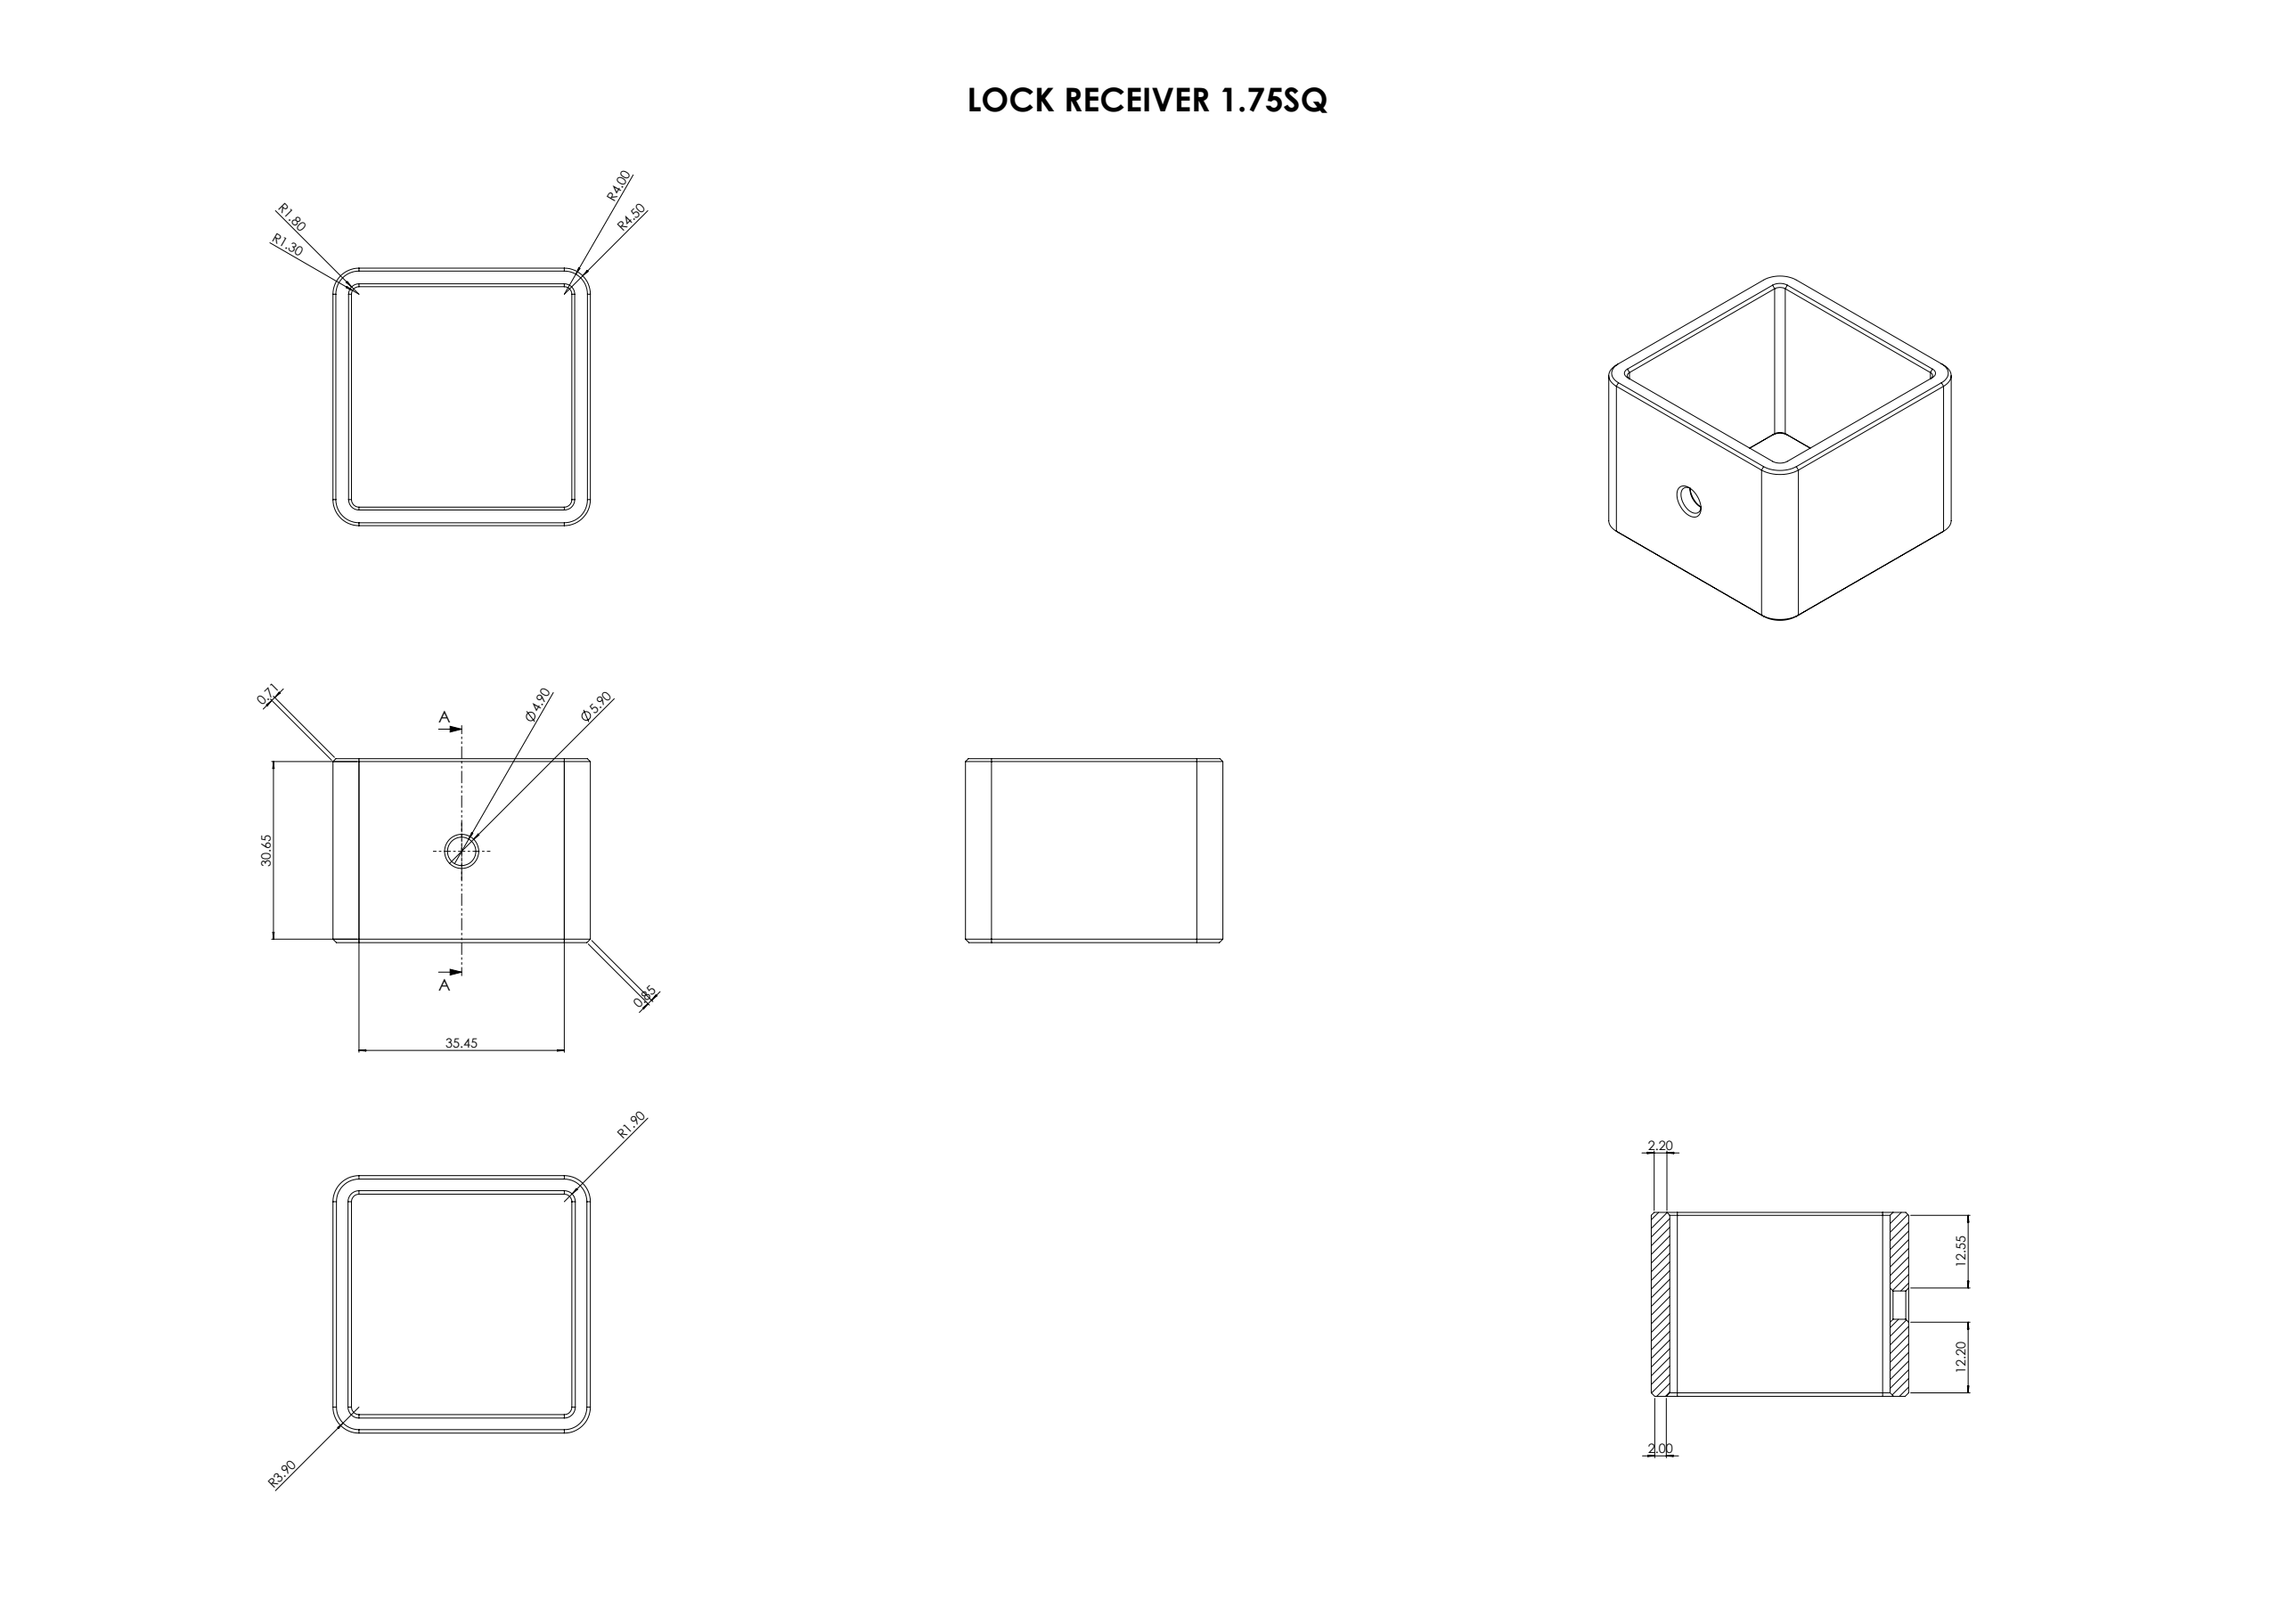
ISO-10303-21;
HEADER;
/* Generated by software containing ST-Developer
 * from STEP Tools, Inc. (www.steptools.com) 
 */

FILE_DESCRIPTION(
/* description */ (''),
/* implementation_level */ '2;1');

FILE_NAME(
/* name */ '04_Lock_Receiver_1.75sq.step',
/* time_stamp */ '2026-10-25T01:30:15-07:00',
/* author */ (''),
/* organization */ (''),
/* preprocessor_version */ 'ST-DEVELOPER v20.2',
/* originating_system */ 'Autodesk Translation Framework v15.15.0.0',
/* authorisation */ '');

FILE_SCHEMA (('AUTOMOTIVE_DESIGN { 1 0 10303 214 3 1 1 }'));
ENDSEC;

DATA;
#10=MECHANICAL_DESIGN_GEOMETRIC_PRESENTATION_REPRESENTATION('',(#566),#32309);
#538=SHAPE_REPRESENTATION_RELATIONSHIP('SRR','None',#32365,#552);
#552=ADVANCED_BREP_SHAPE_REPRESENTATION('',(#580),#32298);
#566=STYLED_ITEM('',(#32516),#580);
#580=MANIFOLD_SOLID_BREP('Body1',#13807);
#595=FACE_BOUND('',#2179,.T.);
#596=FACE_BOUND('',#2182,.T.);
#597=FACE_BOUND('',#2196,.T.);
#598=FACE_BOUND('',#2218,.T.);
#676=CYLINDRICAL_SURFACE('',#14118,2.45);
#677=CYLINDRICAL_SURFACE('',#14140,1.30000000000001);
#678=CYLINDRICAL_SURFACE('',#14143,1.30000000000001);
#679=CYLINDRICAL_SURFACE('',#14164,4.50000000000001);
#680=CYLINDRICAL_SURFACE('',#14167,4.50000000000001);
#681=CYLINDRICAL_SURFACE('',#14198,1.3);
#682=CYLINDRICAL_SURFACE('',#14199,1.3);
#683=CYLINDRICAL_SURFACE('',#14201,4.5);
#684=CYLINDRICAL_SURFACE('',#14203,4.5);
#819=CIRCLE('',#14116,2.95);
#820=CIRCLE('',#14117,2.45);
#821=CIRCLE('',#14119,2.45);
#822=CIRCLE('',#14122,2.95);
#823=CIRCLE('',#14126,1.80000000000001);
#824=CIRCLE('',#14127,1.30000000000001);
#825=CIRCLE('',#14130,1.80000000000001);
#826=CIRCLE('',#14131,1.30000000000001);
#827=CIRCLE('',#14134,1.8);
#828=CIRCLE('',#14135,1.3);
#829=CIRCLE('',#14138,1.8);
#830=CIRCLE('',#14139,1.3);
#831=CIRCLE('',#14141,1.30000000000001);
#832=CIRCLE('',#14144,1.30000000000001);
#833=CIRCLE('',#14147,4.00000000000001);
#834=CIRCLE('',#14148,4.00000000000001);
#835=CIRCLE('',#14149,4.);
#836=CIRCLE('',#14150,4.);
#837=CIRCLE('',#14152,4.50000000000001);
#838=CIRCLE('',#14155,4.50000000000001);
#839=CIRCLE('',#14158,4.5);
#840=CIRCLE('',#14161,4.5);
#841=CIRCLE('',#14165,4.50000000000001);
#842=CIRCLE('',#14168,4.50000000000001);
#843=CIRCLE('',#14171,3.90000000000001);
#844=CIRCLE('',#14174,3.90000000000001);
#845=CIRCLE('',#14177,3.9);
#846=CIRCLE('',#14178,4.5);
#847=CIRCLE('',#14181,3.9);
#848=CIRCLE('',#14182,4.5);
#849=CIRCLE('',#14184,1.90000000000001);
#850=CIRCLE('',#14185,1.9);
#851=CIRCLE('',#14186,1.9);
#852=CIRCLE('',#14187,1.90000000000001);
#853=CIRCLE('',#14192,1.3);
#854=CIRCLE('',#14195,1.3);
#1117=CONICAL_SURFACE('',#14115,2.7,0.785398163397451);
#1118=CONICAL_SURFACE('',#14121,2.7,0.785398163397448);
#1119=CONICAL_SURFACE('',#14125,1.55000000000001,0.785398163397447);
#1120=CONICAL_SURFACE('',#14129,1.55000000000001,0.785398163397447);
#1121=CONICAL_SURFACE('',#14133,1.55,0.785398163397449);
#1122=CONICAL_SURFACE('',#14137,1.55,0.785398163397448);
#1123=CONICAL_SURFACE('',#14151,4.25000000000001,0.785398163397448);
#1124=CONICAL_SURFACE('',#14154,4.25000000000001,0.785398163397448);
#1125=CONICAL_SURFACE('',#14157,4.25,0.785398163397448);
#1126=CONICAL_SURFACE('',#14160,4.25,0.785398163397448);
#1127=CONICAL_SURFACE('',#14170,4.20000000000001,0.78539816339745);
#1128=CONICAL_SURFACE('',#14173,4.20000000000001,0.78539816339745);
#1129=CONICAL_SURFACE('',#14176,4.2,0.785398163397449);
#1130=CONICAL_SURFACE('',#14180,4.2,0.785398163397449);
#1131=CONICAL_SURFACE('',#14189,1.60000000000001,0.785398163397449);
#1132=CONICAL_SURFACE('',#14191,1.6,0.785398163397447);
#1133=CONICAL_SURFACE('',#14194,1.6,0.785398163397448);
#1134=CONICAL_SURFACE('',#14197,1.60000000000001,0.78539816339745);
#1373=FACE_OUTER_BOUND('',#2176,.T.);
#1374=FACE_OUTER_BOUND('',#2177,.T.);
#1375=FACE_OUTER_BOUND('',#2178,.T.);
#1376=FACE_OUTER_BOUND('',#2180,.T.);
#1377=FACE_OUTER_BOUND('',#2181,.T.);
#1378=FACE_OUTER_BOUND('',#2183,.T.);
#1379=FACE_OUTER_BOUND('',#2184,.T.);
#1380=FACE_OUTER_BOUND('',#2185,.T.);
#1381=FACE_OUTER_BOUND('',#2186,.T.);
#1382=FACE_OUTER_BOUND('',#2187,.T.);
#1383=FACE_OUTER_BOUND('',#2188,.T.);
#1384=FACE_OUTER_BOUND('',#2189,.T.);
#1385=FACE_OUTER_BOUND('',#2190,.T.);
#1386=FACE_OUTER_BOUND('',#2191,.T.);
#1387=FACE_OUTER_BOUND('',#2192,.T.);
#1388=FACE_OUTER_BOUND('',#2193,.T.);
#1389=FACE_OUTER_BOUND('',#2194,.T.);
#1390=FACE_OUTER_BOUND('',#2195,.T.);
#1391=FACE_OUTER_BOUND('',#2197,.T.);
#1392=FACE_OUTER_BOUND('',#2198,.T.);
#1393=FACE_OUTER_BOUND('',#2199,.T.);
#1394=FACE_OUTER_BOUND('',#2200,.T.);
#1395=FACE_OUTER_BOUND('',#2201,.T.);
#1396=FACE_OUTER_BOUND('',#2202,.T.);
#1397=FACE_OUTER_BOUND('',#2203,.T.);
#1398=FACE_OUTER_BOUND('',#2204,.T.);
#1399=FACE_OUTER_BOUND('',#2205,.T.);
#1400=FACE_OUTER_BOUND('',#2206,.T.);
#1401=FACE_OUTER_BOUND('',#2207,.T.);
#1402=FACE_OUTER_BOUND('',#2208,.T.);
#1403=FACE_OUTER_BOUND('',#2209,.T.);
#1404=FACE_OUTER_BOUND('',#2210,.T.);
#1405=FACE_OUTER_BOUND('',#2211,.T.);
#1406=FACE_OUTER_BOUND('',#2212,.T.);
#1407=FACE_OUTER_BOUND('',#2213,.T.);
#1408=FACE_OUTER_BOUND('',#2214,.T.);
#1409=FACE_OUTER_BOUND('',#2215,.T.);
#1410=FACE_OUTER_BOUND('',#2216,.T.);
#1411=FACE_OUTER_BOUND('',#2217,.T.);
#1412=FACE_OUTER_BOUND('',#2219,.T.);
#1413=FACE_OUTER_BOUND('',#2220,.T.);
#1414=FACE_OUTER_BOUND('',#2221,.T.);
#1415=FACE_OUTER_BOUND('',#2222,.T.);
#1416=FACE_OUTER_BOUND('',#2223,.T.);
#1417=FACE_OUTER_BOUND('',#2224,.T.);
#1418=FACE_OUTER_BOUND('',#2225,.T.);
#1419=FACE_OUTER_BOUND('',#2226,.T.);
#1420=FACE_OUTER_BOUND('',#2227,.T.);
#1421=FACE_OUTER_BOUND('',#2228,.T.);
#1422=FACE_OUTER_BOUND('',#2229,.T.);
#1423=FACE_OUTER_BOUND('',#2230,.T.);
#1424=FACE_OUTER_BOUND('',#2231,.T.);
#1425=FACE_OUTER_BOUND('',#2232,.T.);
#2176=EDGE_LOOP('',(#9317,#9318,#9319,#9320));
#2177=EDGE_LOOP('',(#9321,#9322,#9323,#9324));
#2178=EDGE_LOOP('',(#9325,#9326,#9327,#9328));
#2179=EDGE_LOOP('',(#9329));
#2180=EDGE_LOOP('',(#9330,#9331,#9332,#9333));
#2181=EDGE_LOOP('',(#9334,#9335,#9336,#9337));
#2182=EDGE_LOOP('',(#9338));
#2183=EDGE_LOOP('',(#9339,#9340,#9341,#9342));
#2184=EDGE_LOOP('',(#9343,#9344,#9345,#9346));
#2185=EDGE_LOOP('',(#9347,#9348,#9349,#9350));
#2186=EDGE_LOOP('',(#9351,#9352,#9353,#9354));
#2187=EDGE_LOOP('',(#9355,#9356,#9357,#9358));
#2188=EDGE_LOOP('',(#9359,#9360,#9361,#9362));
#2189=EDGE_LOOP('',(#9363,#9364,#9365,#9366));
#2190=EDGE_LOOP('',(#9367,#9368,#9369,#9370));
#2191=EDGE_LOOP('',(#9371,#9372,#9373,#9374));
#2192=EDGE_LOOP('',(#9375,#9376,#9377,#9378));
#2193=EDGE_LOOP('',(#9379,#9380,#9381,#9382));
#2194=EDGE_LOOP('',(#9383,#9384,#9385,#9386));
#2195=EDGE_LOOP('',(#9387,#9388,#9389,#9390,#9391,#9392,#9393,#9394));
#2196=EDGE_LOOP('',(#9395,#9396,#9397,#9398,#9399,#9400,#9401,#9402));
#2197=EDGE_LOOP('',(#9403,#9404,#9405,#9406));
#2198=EDGE_LOOP('',(#9407,#9408,#9409,#9410));
#2199=EDGE_LOOP('',(#9411,#9412,#9413,#9414));
#2200=EDGE_LOOP('',(#9415,#9416,#9417,#9418));
#2201=EDGE_LOOP('',(#9419,#9420,#9421,#9422));
#2202=EDGE_LOOP('',(#9423,#9424,#9425,#9426));
#2203=EDGE_LOOP('',(#9427,#9428,#9429,#9430));
#2204=EDGE_LOOP('',(#9431,#9432,#9433,#9434));
#2205=EDGE_LOOP('',(#9435,#9436,#9437,#9438));
#2206=EDGE_LOOP('',(#9439,#9440,#9441,#9442));
#2207=EDGE_LOOP('',(#9443,#9444,#9445,#9446));
#2208=EDGE_LOOP('',(#9447,#9448,#9449,#9450));
#2209=EDGE_LOOP('',(#9451,#9452,#9453,#9454));
#2210=EDGE_LOOP('',(#9455,#9456,#9457,#9458));
#2211=EDGE_LOOP('',(#9459,#9460,#9461,#9462));
#2212=EDGE_LOOP('',(#9463,#9464,#9465,#9466));
#2213=EDGE_LOOP('',(#9467,#9468,#9469,#9470));
#2214=EDGE_LOOP('',(#9471,#9472,#9473,#9474));
#2215=EDGE_LOOP('',(#9475,#9476,#9477,#9478));
#2216=EDGE_LOOP('',(#9479,#9480,#9481,#9482));
#2217=EDGE_LOOP('',(#9483,#9484,#9485,#9486,#9487,#9488,#9489,#9490));
#2218=EDGE_LOOP('',(#9491,#9492,#9493,#9494,#9495,#9496,#9497,#9498));
#2219=EDGE_LOOP('',(#9499,#9500,#9501,#9502));
#2220=EDGE_LOOP('',(#9503,#9504,#9505,#9506));
#2221=EDGE_LOOP('',(#9507,#9508,#9509,#9510));
#2222=EDGE_LOOP('',(#9511,#9512,#9513,#9514));
#2223=EDGE_LOOP('',(#9515,#9516,#9517,#9518));
#2224=EDGE_LOOP('',(#9519,#9520,#9521,#9522));
#2225=EDGE_LOOP('',(#9523,#9524,#9525,#9526));
#2226=EDGE_LOOP('',(#9527,#9528,#9529,#9530));
#2227=EDGE_LOOP('',(#9531,#9532,#9533,#9534));
#2228=EDGE_LOOP('',(#9535,#9536,#9537,#9538));
#2229=EDGE_LOOP('',(#9539,#9540,#9541,#9542));
#2230=EDGE_LOOP('',(#9543,#9544,#9545,#9546));
#2231=EDGE_LOOP('',(#9547,#9548,#9549,#9550));
#2232=EDGE_LOOP('',(#9551,#9552,#9553,#9554));
#3065=LINE('',#21996,#4376);
#3066=LINE('',#22000,#4377);
#3067=LINE('',#22005,#4378);
#3068=LINE('',#22007,#4379);
#3069=LINE('',#22009,#4380);
#3070=LINE('',#22010,#4381);
#3071=LINE('',#22014,#4382);
#3072=LINE('',#22018,#4383);
#3073=LINE('',#22020,#4384);
#3074=LINE('',#22022,#4385);
#3075=LINE('',#22023,#4386);
#3076=LINE('',#22027,#4387);
#3077=LINE('',#22029,#4388);
#3078=LINE('',#22031,#4389);
#3079=LINE('',#22032,#4390);
#3080=LINE('',#22036,#4391);
#3081=LINE('',#22042,#4392);
#3082=LINE('',#22043,#4393);
#3083=LINE('',#22044,#4394);
#3084=LINE('',#22047,#4395);
#3085=LINE('',#22052,#4396);
#3086=LINE('',#22053,#4397);
#3087=LINE('',#22057,#4398);
#3088=LINE('',#22063,#4399);
#3089=LINE('',#22064,#4400);
#3090=LINE('',#22065,#4401);
#3091=LINE('',#22071,#4402);
#3092=LINE('',#22075,#4403);
#3093=LINE('',#22076,#4404);
#3094=LINE('',#22079,#4405);
#3095=LINE('',#22083,#4406);
#3096=LINE('',#22084,#4407);
#3097=LINE('',#22090,#4408);
#3098=LINE('',#22094,#4409);
#3099=LINE('',#22098,#4410);
#3100=LINE('',#22101,#4411);
#3101=LINE('',#22104,#4412);
#3102=LINE('',#22105,#4413);
#3103=LINE('',#22109,#4414);
#3104=LINE('',#22110,#4415);
#3105=LINE('',#22113,#4416);
#3106=LINE('',#22117,#4417);
#3107=LINE('',#22118,#4418);
#3108=LINE('',#22121,#4419);
#3109=LINE('',#22125,#4420);
#3110=LINE('',#22126,#4421);
#3111=LINE('',#22128,#4422);
#3112=LINE('',#22133,#4423);
#3113=LINE('',#22135,#4424);
#3114=LINE('',#22136,#4425);
#3115=LINE('',#22139,#4426);
#3116=LINE('',#22143,#4427);
#3117=LINE('',#22144,#4428);
#3118=LINE('',#22149,#4429);
#3119=LINE('',#22151,#4430);
#3120=LINE('',#22152,#4431);
#3121=LINE('',#22155,#4432);
#3122=LINE('',#22159,#4433);
#3123=LINE('',#22160,#4434);
#3124=LINE('',#22163,#4435);
#3125=LINE('',#22167,#4436);
#3126=LINE('',#22168,#4437);
#3127=LINE('',#22172,#4438);
#3128=LINE('',#22178,#4439);
#3129=LINE('',#22179,#4440);
#3130=LINE('',#22180,#4441);
#3131=LINE('',#22187,#4442);
#3132=LINE('',#22191,#4443);
#3133=LINE('',#22195,#4444);
#3134=LINE('',#22199,#4445);
#3135=LINE('',#22202,#4446);
#3136=LINE('',#22203,#4447);
#3137=LINE('',#22205,#4448);
#3138=LINE('',#22207,#4449);
#3139=LINE('',#22210,#4450);
#3140=LINE('',#22214,#4451);
#3141=LINE('',#22215,#4452);
#3142=LINE('',#22217,#4453);
#3143=LINE('',#22220,#4454);
#3144=LINE('',#22223,#4455);
#3145=LINE('',#22225,#4456);
#3146=LINE('',#22228,#4457);
#3147=LINE('',#22230,#4458);
#4376=VECTOR('',#15461,2.7);
#4377=VECTOR('',#15466,2.45);
#4378=VECTOR('',#15471,10.);
#4379=VECTOR('',#15472,10.);
#4380=VECTOR('',#15473,10.);
#4381=VECTOR('',#15474,10.);
#4382=VECTOR('',#15479,2.7);
#4383=VECTOR('',#15482,10.);
#4384=VECTOR('',#15483,10.);
#4385=VECTOR('',#15484,10.);
#4386=VECTOR('',#15485,10.);
#4387=VECTOR('',#15488,10.);
#4388=VECTOR('',#15489,10.);
#4389=VECTOR('',#15490,10.);
#4390=VECTOR('',#15491,10.);
#4391=VECTOR('',#15494,10.);
#4392=VECTOR('',#15501,10.);
#4393=VECTOR('',#15502,10.);
#4394=VECTOR('',#15503,10.);
#4395=VECTOR('',#15506,10.);
#4396=VECTOR('',#15513,10.);
#4397=VECTOR('',#15514,10.);
#4398=VECTOR('',#15517,10.);
#4399=VECTOR('',#15524,10.);
#4400=VECTOR('',#15525,10.);
#4401=VECTOR('',#15526,10.);
#4402=VECTOR('',#15535,10.);
#4403=VECTOR('',#15540,10.);
#4404=VECTOR('',#15541,10.);
#4405=VECTOR('',#15544,10.);
#4406=VECTOR('',#15549,10.);
#4407=VECTOR('',#15550,10.);
#4408=VECTOR('',#15555,10.);
#4409=VECTOR('',#15558,10.);
#4410=VECTOR('',#15561,10.);
#4411=VECTOR('',#15564,10.);
#4412=VECTOR('',#15567,10.);
#4413=VECTOR('',#15568,10.);
#4414=VECTOR('',#15573,10.);
#4415=VECTOR('',#15574,10.);
#4416=VECTOR('',#15577,10.);
#4417=VECTOR('',#15582,10.);
#4418=VECTOR('',#15583,10.);
#4419=VECTOR('',#15586,10.);
#4420=VECTOR('',#15591,10.);
#4421=VECTOR('',#15592,10.);
#4422=VECTOR('',#15595,10.);
#4423=VECTOR('',#15602,10.);
#4424=VECTOR('',#15603,10.);
#4425=VECTOR('',#15604,10.);
#4426=VECTOR('',#15607,10.);
#4427=VECTOR('',#15612,10.);
#4428=VECTOR('',#15613,10.);
#4429=VECTOR('',#15620,10.);
#4430=VECTOR('',#15621,10.);
#4431=VECTOR('',#15622,10.);
#4432=VECTOR('',#15625,10.);
#4433=VECTOR('',#15630,10.);
#4434=VECTOR('',#15631,10.);
#4435=VECTOR('',#15634,10.);
#4436=VECTOR('',#15639,10.);
#4437=VECTOR('',#15640,10.);
#4438=VECTOR('',#15643,10.);
#4439=VECTOR('',#15650,10.);
#4440=VECTOR('',#15651,10.);
#4441=VECTOR('',#15652,10.);
#4442=VECTOR('',#15661,10.);
#4443=VECTOR('',#15664,10.);
#4444=VECTOR('',#15667,10.);
#4445=VECTOR('',#15670,10.);
#4446=VECTOR('',#15675,10.);
#4447=VECTOR('',#15676,10.);
#4448=VECTOR('',#15679,10.);
#4449=VECTOR('',#15682,10.);
#4450=VECTOR('',#15685,10.);
#4451=VECTOR('',#15690,10.);
#4452=VECTOR('',#15691,10.);
#4453=VECTOR('',#15694,10.);
#4454=VECTOR('',#15699,10.);
#4455=VECTOR('',#15704,10.);
#4456=VECTOR('',#15707,10.);
#4457=VECTOR('',#15712,10.);
#4458=VECTOR('',#15715,10.);
#5712=VERTEX_POINT('',#21993);
#5713=VERTEX_POINT('',#21995);
#5714=VERTEX_POINT('',#21999);
#5715=VERTEX_POINT('',#22003);
#5716=VERTEX_POINT('',#22004);
#5717=VERTEX_POINT('',#22006);
#5718=VERTEX_POINT('',#22008);
#5719=VERTEX_POINT('',#22012);
#5720=VERTEX_POINT('',#22016);
#5721=VERTEX_POINT('',#22017);
#5722=VERTEX_POINT('',#22019);
#5723=VERTEX_POINT('',#22021);
#5724=VERTEX_POINT('',#22025);
#5725=VERTEX_POINT('',#22026);
#5726=VERTEX_POINT('',#22028);
#5727=VERTEX_POINT('',#22030);
#5728=VERTEX_POINT('',#22034);
#5729=VERTEX_POINT('',#22035);
#5730=VERTEX_POINT('',#22040);
#5731=VERTEX_POINT('',#22041);
#5732=VERTEX_POINT('',#22046);
#5733=VERTEX_POINT('',#22051);
#5734=VERTEX_POINT('',#22055);
#5735=VERTEX_POINT('',#22056);
#5736=VERTEX_POINT('',#22061);
#5737=VERTEX_POINT('',#22062);
#5738=VERTEX_POINT('',#22070);
#5739=VERTEX_POINT('',#22074);
#5740=VERTEX_POINT('',#22078);
#5741=VERTEX_POINT('',#22082);
#5742=VERTEX_POINT('',#22086);
#5743=VERTEX_POINT('',#22087);
#5744=VERTEX_POINT('',#22089);
#5745=VERTEX_POINT('',#22091);
#5746=VERTEX_POINT('',#22093);
#5747=VERTEX_POINT('',#22095);
#5748=VERTEX_POINT('',#22097);
#5749=VERTEX_POINT('',#22099);
#5750=VERTEX_POINT('',#22103);
#5751=VERTEX_POINT('',#22108);
#5752=VERTEX_POINT('',#22112);
#5753=VERTEX_POINT('',#22116);
#5754=VERTEX_POINT('',#22120);
#5755=VERTEX_POINT('',#22124);
#5756=VERTEX_POINT('',#22132);
#5757=VERTEX_POINT('',#22134);
#5758=VERTEX_POINT('',#22138);
#5759=VERTEX_POINT('',#22142);
#5760=VERTEX_POINT('',#22148);
#5761=VERTEX_POINT('',#22150);
#5762=VERTEX_POINT('',#22154);
#5763=VERTEX_POINT('',#22158);
#5764=VERTEX_POINT('',#22162);
#5765=VERTEX_POINT('',#22166);
#5766=VERTEX_POINT('',#22170);
#5767=VERTEX_POINT('',#22171);
#5768=VERTEX_POINT('',#22176);
#5769=VERTEX_POINT('',#22177);
#5770=VERTEX_POINT('',#22185);
#5771=VERTEX_POINT('',#22186);
#5772=VERTEX_POINT('',#22188);
#5773=VERTEX_POINT('',#22190);
#5774=VERTEX_POINT('',#22192);
#5775=VERTEX_POINT('',#22194);
#5776=VERTEX_POINT('',#22196);
#5777=VERTEX_POINT('',#22198);
#5778=VERTEX_POINT('',#22209);
#5779=VERTEX_POINT('',#22213);
#7035=EDGE_CURVE('',#5712,#5712,#819,.T.);
#7036=EDGE_CURVE('',#5712,#5713,#3065,.T.);
#7037=EDGE_CURVE('',#5713,#5713,#820,.T.);
#7038=EDGE_CURVE('',#5713,#5714,#3066,.T.);
#7039=EDGE_CURVE('',#5714,#5714,#821,.T.);
#7040=EDGE_CURVE('',#5715,#5716,#3067,.T.);
#7041=EDGE_CURVE('',#5715,#5717,#3068,.T.);
#7042=EDGE_CURVE('',#5718,#5717,#3069,.T.);
#7043=EDGE_CURVE('',#5716,#5718,#3070,.T.);
#7044=EDGE_CURVE('',#5719,#5719,#822,.T.);
#7045=EDGE_CURVE('',#5719,#5714,#3071,.T.);
#7046=EDGE_CURVE('',#5720,#5721,#3072,.T.);
#7047=EDGE_CURVE('',#5720,#5722,#3073,.T.);
#7048=EDGE_CURVE('',#5723,#5722,#3074,.T.);
#7049=EDGE_CURVE('',#5721,#5723,#3075,.T.);
#7050=EDGE_CURVE('',#5724,#5725,#3076,.T.);
#7051=EDGE_CURVE('',#5725,#5726,#3077,.T.);
#7052=EDGE_CURVE('',#5726,#5727,#3078,.T.);
#7053=EDGE_CURVE('',#5727,#5724,#3079,.T.);
#7054=EDGE_CURVE('',#5728,#5729,#3080,.T.);
#7055=EDGE_CURVE('',#5729,#5725,#823,.T.);
#7056=EDGE_CURVE('',#5724,#5728,#824,.T.);
#7057=EDGE_CURVE('',#5730,#5731,#3081,.T.);
#7058=EDGE_CURVE('',#5731,#5729,#3082,.T.);
#7059=EDGE_CURVE('',#5728,#5730,#3083,.T.);
#7060=EDGE_CURVE('',#5720,#5732,#3084,.T.);
#7061=EDGE_CURVE('',#5732,#5731,#825,.T.);
#7062=EDGE_CURVE('',#5730,#5720,#826,.T.);
#7063=EDGE_CURVE('',#5721,#5733,#3085,.T.);
#7064=EDGE_CURVE('',#5733,#5732,#3086,.T.);
#7065=EDGE_CURVE('',#5734,#5735,#3087,.T.);
#7066=EDGE_CURVE('',#5735,#5733,#827,.T.);
#7067=EDGE_CURVE('',#5721,#5734,#828,.T.);
#7068=EDGE_CURVE('',#5736,#5737,#3088,.T.);
#7069=EDGE_CURVE('',#5737,#5735,#3089,.T.);
#7070=EDGE_CURVE('',#5734,#5736,#3090,.T.);
#7071=EDGE_CURVE('',#5726,#5737,#829,.T.);
#7072=EDGE_CURVE('',#5736,#5727,#830,.T.);
#7073=EDGE_CURVE('',#5730,#5738,#3091,.T.);
#7074=EDGE_CURVE('',#5722,#5738,#831,.T.);
#7075=EDGE_CURVE('',#5728,#5739,#3092,.T.);
#7076=EDGE_CURVE('',#5738,#5739,#3093,.T.);
#7077=EDGE_CURVE('',#5724,#5740,#3094,.T.);
#7078=EDGE_CURVE('',#5739,#5740,#832,.T.);
#7079=EDGE_CURVE('',#5727,#5741,#3095,.T.);
#7080=EDGE_CURVE('',#5740,#5741,#3096,.T.);
#7081=EDGE_CURVE('',#5742,#5743,#833,.T.);
#7082=EDGE_CURVE('',#5744,#5742,#3097,.T.);
#7083=EDGE_CURVE('',#5745,#5744,#834,.T.);
#7084=EDGE_CURVE('',#5746,#5745,#3098,.T.);
#7085=EDGE_CURVE('',#5747,#5746,#835,.T.);
#7086=EDGE_CURVE('',#5748,#5747,#3099,.T.);
#7087=EDGE_CURVE('',#5749,#5748,#836,.T.);
#7088=EDGE_CURVE('',#5743,#5749,#3100,.T.);
#7089=EDGE_CURVE('',#5750,#5742,#3101,.T.);
#7090=EDGE_CURVE('',#5743,#5716,#3102,.T.);
#7091=EDGE_CURVE('',#5716,#5750,#837,.T.);
#7092=EDGE_CURVE('',#5750,#5751,#3103,.T.);
#7093=EDGE_CURVE('',#5751,#5744,#3104,.T.);
#7094=EDGE_CURVE('',#5752,#5745,#3105,.T.);
#7095=EDGE_CURVE('',#5751,#5752,#838,.T.);
#7096=EDGE_CURVE('',#5752,#5753,#3106,.T.);
#7097=EDGE_CURVE('',#5753,#5746,#3107,.T.);
#7098=EDGE_CURVE('',#5754,#5747,#3108,.T.);
#7099=EDGE_CURVE('',#5753,#5754,#839,.T.);
#7100=EDGE_CURVE('',#5754,#5755,#3109,.T.);
#7101=EDGE_CURVE('',#5755,#5748,#3110,.T.);
#7102=EDGE_CURVE('',#5715,#5749,#3111,.T.);
#7103=EDGE_CURVE('',#5755,#5715,#840,.T.);
#7104=EDGE_CURVE('',#5752,#5756,#3112,.T.);
#7105=EDGE_CURVE('',#5757,#5756,#3113,.T.);
#7106=EDGE_CURVE('',#5753,#5757,#3114,.T.);
#7107=EDGE_CURVE('',#5751,#5758,#3115,.T.);
#7108=EDGE_CURVE('',#5756,#5758,#841,.T.);
#7109=EDGE_CURVE('',#5750,#5759,#3116,.T.);
#7110=EDGE_CURVE('',#5758,#5759,#3117,.T.);
#7111=EDGE_CURVE('',#5759,#5718,#842,.T.);
#7112=EDGE_CURVE('',#5756,#5760,#3118,.T.);
#7113=EDGE_CURVE('',#5760,#5761,#3119,.T.);
#7114=EDGE_CURVE('',#5761,#5757,#3120,.T.);
#7115=EDGE_CURVE('',#5758,#5762,#3121,.T.);
#7116=EDGE_CURVE('',#5762,#5760,#843,.T.);
#7117=EDGE_CURVE('',#5759,#5763,#3122,.T.);
#7118=EDGE_CURVE('',#5763,#5762,#3123,.T.);
#7119=EDGE_CURVE('',#5718,#5764,#3124,.T.);
#7120=EDGE_CURVE('',#5764,#5763,#844,.T.);
#7121=EDGE_CURVE('',#5717,#5765,#3125,.T.);
#7122=EDGE_CURVE('',#5765,#5764,#3126,.T.);
#7123=EDGE_CURVE('',#5766,#5767,#3127,.T.);
#7124=EDGE_CURVE('',#5767,#5765,#845,.T.);
#7125=EDGE_CURVE('',#5717,#5766,#846,.T.);
#7126=EDGE_CURVE('',#5768,#5769,#3128,.T.);
#7127=EDGE_CURVE('',#5769,#5767,#3129,.T.);
#7128=EDGE_CURVE('',#5766,#5768,#3130,.T.);
#7129=EDGE_CURVE('',#5761,#5769,#847,.T.);
#7130=EDGE_CURVE('',#5768,#5757,#848,.T.);
#7131=EDGE_CURVE('',#5770,#5771,#3131,.T.);
#7132=EDGE_CURVE('',#5772,#5770,#849,.T.);
#7133=EDGE_CURVE('',#5773,#5772,#3132,.T.);
#7134=EDGE_CURVE('',#5774,#5773,#850,.T.);
#7135=EDGE_CURVE('',#5775,#5774,#3133,.T.);
#7136=EDGE_CURVE('',#5776,#5775,#851,.T.);
#7137=EDGE_CURVE('',#5777,#5776,#3134,.T.);
#7138=EDGE_CURVE('',#5771,#5777,#852,.T.);
#7139=EDGE_CURVE('',#5739,#5770,#3135,.T.);
#7140=EDGE_CURVE('',#5771,#5738,#3136,.T.);
#7141=EDGE_CURVE('',#5740,#5772,#3137,.T.);
#7142=EDGE_CURVE('',#5741,#5773,#3138,.T.);
#7143=EDGE_CURVE('',#5778,#5774,#3139,.T.);
#7144=EDGE_CURVE('',#5741,#5778,#853,.T.);
#7145=EDGE_CURVE('',#5779,#5775,#3140,.T.);
#7146=EDGE_CURVE('',#5778,#5779,#3141,.T.);
#7147=EDGE_CURVE('',#5723,#5776,#3142,.T.);
#7148=EDGE_CURVE('',#5779,#5723,#854,.T.);
#7149=EDGE_CURVE('',#5722,#5777,#3143,.T.);
#7150=EDGE_CURVE('',#5736,#5778,#3144,.T.);
#7151=EDGE_CURVE('',#5734,#5779,#3145,.T.);
#7152=EDGE_CURVE('',#5754,#5768,#3146,.T.);
#7153=EDGE_CURVE('',#5755,#5766,#3147,.T.);
#9317=ORIENTED_EDGE('',*,*,#7035,.T.);
#9318=ORIENTED_EDGE('',*,*,#7036,.T.);
#9319=ORIENTED_EDGE('',*,*,#7037,.T.);
#9320=ORIENTED_EDGE('',*,*,#7036,.F.);
#9321=ORIENTED_EDGE('',*,*,#7037,.F.);
#9322=ORIENTED_EDGE('',*,*,#7038,.T.);
#9323=ORIENTED_EDGE('',*,*,#7039,.F.);
#9324=ORIENTED_EDGE('',*,*,#7038,.F.);
#9325=ORIENTED_EDGE('',*,*,#7040,.F.);
#9326=ORIENTED_EDGE('',*,*,#7041,.T.);
#9327=ORIENTED_EDGE('',*,*,#7042,.F.);
#9328=ORIENTED_EDGE('',*,*,#7043,.F.);
#9329=ORIENTED_EDGE('',*,*,#7035,.F.);
#9330=ORIENTED_EDGE('',*,*,#7044,.T.);
#9331=ORIENTED_EDGE('',*,*,#7045,.T.);
#9332=ORIENTED_EDGE('',*,*,#7039,.T.);
#9333=ORIENTED_EDGE('',*,*,#7045,.F.);
#9334=ORIENTED_EDGE('',*,*,#7046,.F.);
#9335=ORIENTED_EDGE('',*,*,#7047,.T.);
#9336=ORIENTED_EDGE('',*,*,#7048,.F.);
#9337=ORIENTED_EDGE('',*,*,#7049,.F.);
#9338=ORIENTED_EDGE('',*,*,#7044,.F.);
#9339=ORIENTED_EDGE('',*,*,#7050,.T.);
#9340=ORIENTED_EDGE('',*,*,#7051,.T.);
#9341=ORIENTED_EDGE('',*,*,#7052,.T.);
#9342=ORIENTED_EDGE('',*,*,#7053,.T.);
#9343=ORIENTED_EDGE('',*,*,#7054,.T.);
#9344=ORIENTED_EDGE('',*,*,#7055,.T.);
#9345=ORIENTED_EDGE('',*,*,#7050,.F.);
#9346=ORIENTED_EDGE('',*,*,#7056,.T.);
#9347=ORIENTED_EDGE('',*,*,#7057,.T.);
#9348=ORIENTED_EDGE('',*,*,#7058,.T.);
#9349=ORIENTED_EDGE('',*,*,#7054,.F.);
#9350=ORIENTED_EDGE('',*,*,#7059,.T.);
#9351=ORIENTED_EDGE('',*,*,#7060,.T.);
#9352=ORIENTED_EDGE('',*,*,#7061,.T.);
#9353=ORIENTED_EDGE('',*,*,#7057,.F.);
#9354=ORIENTED_EDGE('',*,*,#7062,.T.);
#9355=ORIENTED_EDGE('',*,*,#7063,.T.);
#9356=ORIENTED_EDGE('',*,*,#7064,.T.);
#9357=ORIENTED_EDGE('',*,*,#7060,.F.);
#9358=ORIENTED_EDGE('',*,*,#7046,.T.);
#9359=ORIENTED_EDGE('',*,*,#7065,.T.);
#9360=ORIENTED_EDGE('',*,*,#7066,.T.);
#9361=ORIENTED_EDGE('',*,*,#7063,.F.);
#9362=ORIENTED_EDGE('',*,*,#7067,.T.);
#9363=ORIENTED_EDGE('',*,*,#7068,.T.);
#9364=ORIENTED_EDGE('',*,*,#7069,.T.);
#9365=ORIENTED_EDGE('',*,*,#7065,.F.);
#9366=ORIENTED_EDGE('',*,*,#7070,.T.);
#9367=ORIENTED_EDGE('',*,*,#7052,.F.);
#9368=ORIENTED_EDGE('',*,*,#7071,.T.);
#9369=ORIENTED_EDGE('',*,*,#7068,.F.);
#9370=ORIENTED_EDGE('',*,*,#7072,.T.);
#9371=ORIENTED_EDGE('',*,*,#7062,.F.);
#9372=ORIENTED_EDGE('',*,*,#7073,.T.);
#9373=ORIENTED_EDGE('',*,*,#7074,.F.);
#9374=ORIENTED_EDGE('',*,*,#7047,.F.);
#9375=ORIENTED_EDGE('',*,*,#7059,.F.);
#9376=ORIENTED_EDGE('',*,*,#7075,.T.);
#9377=ORIENTED_EDGE('',*,*,#7076,.F.);
#9378=ORIENTED_EDGE('',*,*,#7073,.F.);
#9379=ORIENTED_EDGE('',*,*,#7056,.F.);
#9380=ORIENTED_EDGE('',*,*,#7077,.T.);
#9381=ORIENTED_EDGE('',*,*,#7078,.F.);
#9382=ORIENTED_EDGE('',*,*,#7075,.F.);
#9383=ORIENTED_EDGE('',*,*,#7053,.F.);
#9384=ORIENTED_EDGE('',*,*,#7079,.T.);
#9385=ORIENTED_EDGE('',*,*,#7080,.F.);
#9386=ORIENTED_EDGE('',*,*,#7077,.F.);
#9387=ORIENTED_EDGE('',*,*,#7081,.F.);
#9388=ORIENTED_EDGE('',*,*,#7082,.F.);
#9389=ORIENTED_EDGE('',*,*,#7083,.F.);
#9390=ORIENTED_EDGE('',*,*,#7084,.F.);
#9391=ORIENTED_EDGE('',*,*,#7085,.F.);
#9392=ORIENTED_EDGE('',*,*,#7086,.F.);
#9393=ORIENTED_EDGE('',*,*,#7087,.F.);
#9394=ORIENTED_EDGE('',*,*,#7088,.F.);
#9395=ORIENTED_EDGE('',*,*,#7051,.F.);
#9396=ORIENTED_EDGE('',*,*,#7055,.F.);
#9397=ORIENTED_EDGE('',*,*,#7058,.F.);
#9398=ORIENTED_EDGE('',*,*,#7061,.F.);
#9399=ORIENTED_EDGE('',*,*,#7064,.F.);
#9400=ORIENTED_EDGE('',*,*,#7066,.F.);
#9401=ORIENTED_EDGE('',*,*,#7069,.F.);
#9402=ORIENTED_EDGE('',*,*,#7071,.F.);
#9403=ORIENTED_EDGE('',*,*,#7089,.T.);
#9404=ORIENTED_EDGE('',*,*,#7081,.T.);
#9405=ORIENTED_EDGE('',*,*,#7090,.T.);
#9406=ORIENTED_EDGE('',*,*,#7091,.T.);
#9407=ORIENTED_EDGE('',*,*,#7089,.F.);
#9408=ORIENTED_EDGE('',*,*,#7092,.T.);
#9409=ORIENTED_EDGE('',*,*,#7093,.T.);
#9410=ORIENTED_EDGE('',*,*,#7082,.T.);
#9411=ORIENTED_EDGE('',*,*,#7094,.T.);
#9412=ORIENTED_EDGE('',*,*,#7083,.T.);
#9413=ORIENTED_EDGE('',*,*,#7093,.F.);
#9414=ORIENTED_EDGE('',*,*,#7095,.T.);
#9415=ORIENTED_EDGE('',*,*,#7094,.F.);
#9416=ORIENTED_EDGE('',*,*,#7096,.T.);
#9417=ORIENTED_EDGE('',*,*,#7097,.T.);
#9418=ORIENTED_EDGE('',*,*,#7084,.T.);
#9419=ORIENTED_EDGE('',*,*,#7098,.T.);
#9420=ORIENTED_EDGE('',*,*,#7085,.T.);
#9421=ORIENTED_EDGE('',*,*,#7097,.F.);
#9422=ORIENTED_EDGE('',*,*,#7099,.T.);
#9423=ORIENTED_EDGE('',*,*,#7098,.F.);
#9424=ORIENTED_EDGE('',*,*,#7100,.T.);
#9425=ORIENTED_EDGE('',*,*,#7101,.T.);
#9426=ORIENTED_EDGE('',*,*,#7086,.T.);
#9427=ORIENTED_EDGE('',*,*,#7102,.T.);
#9428=ORIENTED_EDGE('',*,*,#7087,.T.);
#9429=ORIENTED_EDGE('',*,*,#7101,.F.);
#9430=ORIENTED_EDGE('',*,*,#7103,.T.);
#9431=ORIENTED_EDGE('',*,*,#7102,.F.);
#9432=ORIENTED_EDGE('',*,*,#7040,.T.);
#9433=ORIENTED_EDGE('',*,*,#7090,.F.);
#9434=ORIENTED_EDGE('',*,*,#7088,.T.);
#9435=ORIENTED_EDGE('',*,*,#7096,.F.);
#9436=ORIENTED_EDGE('',*,*,#7104,.T.);
#9437=ORIENTED_EDGE('',*,*,#7105,.F.);
#9438=ORIENTED_EDGE('',*,*,#7106,.F.);
#9439=ORIENTED_EDGE('',*,*,#7095,.F.);
#9440=ORIENTED_EDGE('',*,*,#7107,.T.);
#9441=ORIENTED_EDGE('',*,*,#7108,.F.);
#9442=ORIENTED_EDGE('',*,*,#7104,.F.);
#9443=ORIENTED_EDGE('',*,*,#7092,.F.);
#9444=ORIENTED_EDGE('',*,*,#7109,.T.);
#9445=ORIENTED_EDGE('',*,*,#7110,.F.);
#9446=ORIENTED_EDGE('',*,*,#7107,.F.);
#9447=ORIENTED_EDGE('',*,*,#7091,.F.);
#9448=ORIENTED_EDGE('',*,*,#7043,.T.);
#9449=ORIENTED_EDGE('',*,*,#7111,.F.);
#9450=ORIENTED_EDGE('',*,*,#7109,.F.);
#9451=ORIENTED_EDGE('',*,*,#7112,.T.);
#9452=ORIENTED_EDGE('',*,*,#7113,.T.);
#9453=ORIENTED_EDGE('',*,*,#7114,.T.);
#9454=ORIENTED_EDGE('',*,*,#7105,.T.);
#9455=ORIENTED_EDGE('',*,*,#7115,.T.);
#9456=ORIENTED_EDGE('',*,*,#7116,.T.);
#9457=ORIENTED_EDGE('',*,*,#7112,.F.);
#9458=ORIENTED_EDGE('',*,*,#7108,.T.);
#9459=ORIENTED_EDGE('',*,*,#7117,.T.);
#9460=ORIENTED_EDGE('',*,*,#7118,.T.);
#9461=ORIENTED_EDGE('',*,*,#7115,.F.);
#9462=ORIENTED_EDGE('',*,*,#7110,.T.);
#9463=ORIENTED_EDGE('',*,*,#7119,.T.);
#9464=ORIENTED_EDGE('',*,*,#7120,.T.);
#9465=ORIENTED_EDGE('',*,*,#7117,.F.);
#9466=ORIENTED_EDGE('',*,*,#7111,.T.);
#9467=ORIENTED_EDGE('',*,*,#7121,.T.);
#9468=ORIENTED_EDGE('',*,*,#7122,.T.);
#9469=ORIENTED_EDGE('',*,*,#7119,.F.);
#9470=ORIENTED_EDGE('',*,*,#7042,.T.);
#9471=ORIENTED_EDGE('',*,*,#7123,.T.);
#9472=ORIENTED_EDGE('',*,*,#7124,.T.);
#9473=ORIENTED_EDGE('',*,*,#7121,.F.);
#9474=ORIENTED_EDGE('',*,*,#7125,.T.);
#9475=ORIENTED_EDGE('',*,*,#7126,.T.);
#9476=ORIENTED_EDGE('',*,*,#7127,.T.);
#9477=ORIENTED_EDGE('',*,*,#7123,.F.);
#9478=ORIENTED_EDGE('',*,*,#7128,.T.);
#9479=ORIENTED_EDGE('',*,*,#7114,.F.);
#9480=ORIENTED_EDGE('',*,*,#7129,.T.);
#9481=ORIENTED_EDGE('',*,*,#7126,.F.);
#9482=ORIENTED_EDGE('',*,*,#7130,.T.);
#9483=ORIENTED_EDGE('',*,*,#7113,.F.);
#9484=ORIENTED_EDGE('',*,*,#7116,.F.);
#9485=ORIENTED_EDGE('',*,*,#7118,.F.);
#9486=ORIENTED_EDGE('',*,*,#7120,.F.);
#9487=ORIENTED_EDGE('',*,*,#7122,.F.);
#9488=ORIENTED_EDGE('',*,*,#7124,.F.);
#9489=ORIENTED_EDGE('',*,*,#7127,.F.);
#9490=ORIENTED_EDGE('',*,*,#7129,.F.);
#9491=ORIENTED_EDGE('',*,*,#7131,.F.);
#9492=ORIENTED_EDGE('',*,*,#7132,.F.);
#9493=ORIENTED_EDGE('',*,*,#7133,.F.);
#9494=ORIENTED_EDGE('',*,*,#7134,.F.);
#9495=ORIENTED_EDGE('',*,*,#7135,.F.);
#9496=ORIENTED_EDGE('',*,*,#7136,.F.);
#9497=ORIENTED_EDGE('',*,*,#7137,.F.);
#9498=ORIENTED_EDGE('',*,*,#7138,.F.);
#9499=ORIENTED_EDGE('',*,*,#7139,.T.);
#9500=ORIENTED_EDGE('',*,*,#7131,.T.);
#9501=ORIENTED_EDGE('',*,*,#7140,.T.);
#9502=ORIENTED_EDGE('',*,*,#7076,.T.);
#9503=ORIENTED_EDGE('',*,*,#7141,.T.);
#9504=ORIENTED_EDGE('',*,*,#7132,.T.);
#9505=ORIENTED_EDGE('',*,*,#7139,.F.);
#9506=ORIENTED_EDGE('',*,*,#7078,.T.);
#9507=ORIENTED_EDGE('',*,*,#7142,.T.);
#9508=ORIENTED_EDGE('',*,*,#7133,.T.);
#9509=ORIENTED_EDGE('',*,*,#7141,.F.);
#9510=ORIENTED_EDGE('',*,*,#7080,.T.);
#9511=ORIENTED_EDGE('',*,*,#7143,.T.);
#9512=ORIENTED_EDGE('',*,*,#7134,.T.);
#9513=ORIENTED_EDGE('',*,*,#7142,.F.);
#9514=ORIENTED_EDGE('',*,*,#7144,.T.);
#9515=ORIENTED_EDGE('',*,*,#7145,.T.);
#9516=ORIENTED_EDGE('',*,*,#7135,.T.);
#9517=ORIENTED_EDGE('',*,*,#7143,.F.);
#9518=ORIENTED_EDGE('',*,*,#7146,.T.);
#9519=ORIENTED_EDGE('',*,*,#7147,.T.);
#9520=ORIENTED_EDGE('',*,*,#7136,.T.);
#9521=ORIENTED_EDGE('',*,*,#7145,.F.);
#9522=ORIENTED_EDGE('',*,*,#7148,.T.);
#9523=ORIENTED_EDGE('',*,*,#7149,.T.);
#9524=ORIENTED_EDGE('',*,*,#7137,.T.);
#9525=ORIENTED_EDGE('',*,*,#7147,.F.);
#9526=ORIENTED_EDGE('',*,*,#7048,.T.);
#9527=ORIENTED_EDGE('',*,*,#7140,.F.);
#9528=ORIENTED_EDGE('',*,*,#7138,.T.);
#9529=ORIENTED_EDGE('',*,*,#7149,.F.);
#9530=ORIENTED_EDGE('',*,*,#7074,.T.);
#9531=ORIENTED_EDGE('',*,*,#7072,.F.);
#9532=ORIENTED_EDGE('',*,*,#7150,.T.);
#9533=ORIENTED_EDGE('',*,*,#7144,.F.);
#9534=ORIENTED_EDGE('',*,*,#7079,.F.);
#9535=ORIENTED_EDGE('',*,*,#7067,.F.);
#9536=ORIENTED_EDGE('',*,*,#7049,.T.);
#9537=ORIENTED_EDGE('',*,*,#7148,.F.);
#9538=ORIENTED_EDGE('',*,*,#7151,.F.);
#9539=ORIENTED_EDGE('',*,*,#7070,.F.);
#9540=ORIENTED_EDGE('',*,*,#7151,.T.);
#9541=ORIENTED_EDGE('',*,*,#7146,.F.);
#9542=ORIENTED_EDGE('',*,*,#7150,.F.);
#9543=ORIENTED_EDGE('',*,*,#7099,.F.);
#9544=ORIENTED_EDGE('',*,*,#7106,.T.);
#9545=ORIENTED_EDGE('',*,*,#7130,.F.);
#9546=ORIENTED_EDGE('',*,*,#7152,.F.);
#9547=ORIENTED_EDGE('',*,*,#7100,.F.);
#9548=ORIENTED_EDGE('',*,*,#7152,.T.);
#9549=ORIENTED_EDGE('',*,*,#7128,.F.);
#9550=ORIENTED_EDGE('',*,*,#7153,.F.);
#9551=ORIENTED_EDGE('',*,*,#7103,.F.);
#9552=ORIENTED_EDGE('',*,*,#7153,.T.);
#9553=ORIENTED_EDGE('',*,*,#7125,.F.);
#9554=ORIENTED_EDGE('',*,*,#7041,.F.);
#12647=PLANE('',#14120);
#12648=PLANE('',#14123);
#12649=PLANE('',#14124);
#12650=PLANE('',#14128);
#12651=PLANE('',#14132);
#12652=PLANE('',#14136);
#12653=PLANE('',#14142);
#12654=PLANE('',#14145);
#12655=PLANE('',#14146);
#12656=PLANE('',#14153);
#12657=PLANE('',#14156);
#12658=PLANE('',#14159);
#12659=PLANE('',#14162);
#12660=PLANE('',#14163);
#12661=PLANE('',#14166);
#12662=PLANE('',#14169);
#12663=PLANE('',#14172);
#12664=PLANE('',#14175);
#12665=PLANE('',#14179);
#12666=PLANE('',#14183);
#12667=PLANE('',#14188);
#12668=PLANE('',#14190);
#12669=PLANE('',#14193);
#12670=PLANE('',#14196);
#12671=PLANE('',#14200);
#12672=PLANE('',#14202);
#13136=ADVANCED_FACE('',(#1373),#1117,.F.);
#13137=ADVANCED_FACE('',(#1374),#676,.F.);
#13138=ADVANCED_FACE('',(#1375,#595),#12647,.T.);
#13139=ADVANCED_FACE('',(#1376),#1118,.F.);
#13140=ADVANCED_FACE('',(#1377,#596),#12648,.T.);
#13141=ADVANCED_FACE('',(#1378),#12649,.T.);
#13142=ADVANCED_FACE('',(#1379),#1119,.F.);
#13143=ADVANCED_FACE('',(#1380),#12650,.T.);
#13144=ADVANCED_FACE('',(#1381),#1120,.F.);
#13145=ADVANCED_FACE('',(#1382),#12651,.T.);
#13146=ADVANCED_FACE('',(#1383),#1121,.F.);
#13147=ADVANCED_FACE('',(#1384),#12652,.T.);
#13148=ADVANCED_FACE('',(#1385),#1122,.F.);
#13149=ADVANCED_FACE('',(#1386),#677,.F.);
#13150=ADVANCED_FACE('',(#1387),#12653,.T.);
#13151=ADVANCED_FACE('',(#1388),#678,.F.);
#13152=ADVANCED_FACE('',(#1389),#12654,.T.);
#13153=ADVANCED_FACE('',(#1390,#597),#12655,.T.);
#13154=ADVANCED_FACE('',(#1391),#1123,.T.);
#13155=ADVANCED_FACE('',(#1392),#12656,.T.);
#13156=ADVANCED_FACE('',(#1393),#1124,.T.);
#13157=ADVANCED_FACE('',(#1394),#12657,.T.);
#13158=ADVANCED_FACE('',(#1395),#1125,.T.);
#13159=ADVANCED_FACE('',(#1396),#12658,.T.);
#13160=ADVANCED_FACE('',(#1397),#1126,.T.);
#13161=ADVANCED_FACE('',(#1398),#12659,.T.);
#13162=ADVANCED_FACE('',(#1399),#12660,.T.);
#13163=ADVANCED_FACE('',(#1400),#679,.T.);
#13164=ADVANCED_FACE('',(#1401),#12661,.T.);
#13165=ADVANCED_FACE('',(#1402),#680,.T.);
#13166=ADVANCED_FACE('',(#1403),#12662,.T.);
#13167=ADVANCED_FACE('',(#1404),#1127,.T.);
#13168=ADVANCED_FACE('',(#1405),#12663,.T.);
#13169=ADVANCED_FACE('',(#1406),#1128,.T.);
#13170=ADVANCED_FACE('',(#1407),#12664,.T.);
#13171=ADVANCED_FACE('',(#1408),#1129,.T.);
#13172=ADVANCED_FACE('',(#1409),#12665,.T.);
#13173=ADVANCED_FACE('',(#1410),#1130,.T.);
#13174=ADVANCED_FACE('',(#1411,#598),#12666,.F.);
#13175=ADVANCED_FACE('',(#1412),#12667,.T.);
#13176=ADVANCED_FACE('',(#1413),#1131,.F.);
#13177=ADVANCED_FACE('',(#1414),#12668,.T.);
#13178=ADVANCED_FACE('',(#1415),#1132,.F.);
#13179=ADVANCED_FACE('',(#1416),#12669,.T.);
#13180=ADVANCED_FACE('',(#1417),#1133,.F.);
#13181=ADVANCED_FACE('',(#1418),#12670,.T.);
#13182=ADVANCED_FACE('',(#1419),#1134,.F.);
#13183=ADVANCED_FACE('',(#1420),#681,.F.);
#13184=ADVANCED_FACE('',(#1421),#682,.F.);
#13185=ADVANCED_FACE('',(#1422),#12671,.T.);
#13186=ADVANCED_FACE('',(#1423),#683,.T.);
#13187=ADVANCED_FACE('',(#1424),#12672,.T.);
#13188=ADVANCED_FACE('',(#1425),#684,.T.);
#13807=CLOSED_SHELL('',(#13136,#13137,#13138,#13139,#13140,#13141,#13142,
#13143,#13144,#13145,#13146,#13147,#13148,#13149,#13150,#13151,#13152,#13153,
#13154,#13155,#13156,#13157,#13158,#13159,#13160,#13161,#13162,#13163,#13164,
#13165,#13166,#13167,#13168,#13169,#13170,#13171,#13172,#13173,#13174,#13175,
#13176,#13177,#13178,#13179,#13180,#13181,#13182,#13183,#13184,#13185,#13186,
#13187,#13188));
#14114=AXIS2_PLACEMENT_3D('',#21991,#15455,#15456);
#14115=AXIS2_PLACEMENT_3D('',#21992,#15457,#15458);
#14116=AXIS2_PLACEMENT_3D('',#21994,#15459,#15460);
#14117=AXIS2_PLACEMENT_3D('',#21997,#15462,#15463);
#14118=AXIS2_PLACEMENT_3D('',#21998,#15464,#15465);
#14119=AXIS2_PLACEMENT_3D('',#22001,#15467,#15468);
#14120=AXIS2_PLACEMENT_3D('',#22002,#15469,#15470);
#14121=AXIS2_PLACEMENT_3D('',#22011,#15475,#15476);
#14122=AXIS2_PLACEMENT_3D('',#22013,#15477,#15478);
#14123=AXIS2_PLACEMENT_3D('',#22015,#15480,#15481);
#14124=AXIS2_PLACEMENT_3D('',#22024,#15486,#15487);
#14125=AXIS2_PLACEMENT_3D('',#22033,#15492,#15493);
#14126=AXIS2_PLACEMENT_3D('',#22037,#15495,#15496);
#14127=AXIS2_PLACEMENT_3D('',#22038,#15497,#15498);
#14128=AXIS2_PLACEMENT_3D('',#22039,#15499,#15500);
#14129=AXIS2_PLACEMENT_3D('',#22045,#15504,#15505);
#14130=AXIS2_PLACEMENT_3D('',#22048,#15507,#15508);
#14131=AXIS2_PLACEMENT_3D('',#22049,#15509,#15510);
#14132=AXIS2_PLACEMENT_3D('',#22050,#15511,#15512);
#14133=AXIS2_PLACEMENT_3D('',#22054,#15515,#15516);
#14134=AXIS2_PLACEMENT_3D('',#22058,#15518,#15519);
#14135=AXIS2_PLACEMENT_3D('',#22059,#15520,#15521);
#14136=AXIS2_PLACEMENT_3D('',#22060,#15522,#15523);
#14137=AXIS2_PLACEMENT_3D('',#22066,#15527,#15528);
#14138=AXIS2_PLACEMENT_3D('',#22067,#15529,#15530);
#14139=AXIS2_PLACEMENT_3D('',#22068,#15531,#15532);
#14140=AXIS2_PLACEMENT_3D('',#22069,#15533,#15534);
#14141=AXIS2_PLACEMENT_3D('',#22072,#15536,#15537);
#14142=AXIS2_PLACEMENT_3D('',#22073,#15538,#15539);
#14143=AXIS2_PLACEMENT_3D('',#22077,#15542,#15543);
#14144=AXIS2_PLACEMENT_3D('',#22080,#15545,#15546);
#14145=AXIS2_PLACEMENT_3D('',#22081,#15547,#15548);
#14146=AXIS2_PLACEMENT_3D('',#22085,#15551,#15552);
#14147=AXIS2_PLACEMENT_3D('',#22088,#15553,#15554);
#14148=AXIS2_PLACEMENT_3D('',#22092,#15556,#15557);
#14149=AXIS2_PLACEMENT_3D('',#22096,#15559,#15560);
#14150=AXIS2_PLACEMENT_3D('',#22100,#15562,#15563);
#14151=AXIS2_PLACEMENT_3D('',#22102,#15565,#15566);
#14152=AXIS2_PLACEMENT_3D('',#22106,#15569,#15570);
#14153=AXIS2_PLACEMENT_3D('',#22107,#15571,#15572);
#14154=AXIS2_PLACEMENT_3D('',#22111,#15575,#15576);
#14155=AXIS2_PLACEMENT_3D('',#22114,#15578,#15579);
#14156=AXIS2_PLACEMENT_3D('',#22115,#15580,#15581);
#14157=AXIS2_PLACEMENT_3D('',#22119,#15584,#15585);
#14158=AXIS2_PLACEMENT_3D('',#22122,#15587,#15588);
#14159=AXIS2_PLACEMENT_3D('',#22123,#15589,#15590);
#14160=AXIS2_PLACEMENT_3D('',#22127,#15593,#15594);
#14161=AXIS2_PLACEMENT_3D('',#22129,#15596,#15597);
#14162=AXIS2_PLACEMENT_3D('',#22130,#15598,#15599);
#14163=AXIS2_PLACEMENT_3D('',#22131,#15600,#15601);
#14164=AXIS2_PLACEMENT_3D('',#22137,#15605,#15606);
#14165=AXIS2_PLACEMENT_3D('',#22140,#15608,#15609);
#14166=AXIS2_PLACEMENT_3D('',#22141,#15610,#15611);
#14167=AXIS2_PLACEMENT_3D('',#22145,#15614,#15615);
#14168=AXIS2_PLACEMENT_3D('',#22146,#15616,#15617);
#14169=AXIS2_PLACEMENT_3D('',#22147,#15618,#15619);
#14170=AXIS2_PLACEMENT_3D('',#22153,#15623,#15624);
#14171=AXIS2_PLACEMENT_3D('',#22156,#15626,#15627);
#14172=AXIS2_PLACEMENT_3D('',#22157,#15628,#15629);
#14173=AXIS2_PLACEMENT_3D('',#22161,#15632,#15633);
#14174=AXIS2_PLACEMENT_3D('',#22164,#15635,#15636);
#14175=AXIS2_PLACEMENT_3D('',#22165,#15637,#15638);
#14176=AXIS2_PLACEMENT_3D('',#22169,#15641,#15642);
#14177=AXIS2_PLACEMENT_3D('',#22173,#15644,#15645);
#14178=AXIS2_PLACEMENT_3D('',#22174,#15646,#15647);
#14179=AXIS2_PLACEMENT_3D('',#22175,#15648,#15649);
#14180=AXIS2_PLACEMENT_3D('',#22181,#15653,#15654);
#14181=AXIS2_PLACEMENT_3D('',#22182,#15655,#15656);
#14182=AXIS2_PLACEMENT_3D('',#22183,#15657,#15658);
#14183=AXIS2_PLACEMENT_3D('',#22184,#15659,#15660);
#14184=AXIS2_PLACEMENT_3D('',#22189,#15662,#15663);
#14185=AXIS2_PLACEMENT_3D('',#22193,#15665,#15666);
#14186=AXIS2_PLACEMENT_3D('',#22197,#15668,#15669);
#14187=AXIS2_PLACEMENT_3D('',#22200,#15671,#15672);
#14188=AXIS2_PLACEMENT_3D('',#22201,#15673,#15674);
#14189=AXIS2_PLACEMENT_3D('',#22204,#15677,#15678);
#14190=AXIS2_PLACEMENT_3D('',#22206,#15680,#15681);
#14191=AXIS2_PLACEMENT_3D('',#22208,#15683,#15684);
#14192=AXIS2_PLACEMENT_3D('',#22211,#15686,#15687);
#14193=AXIS2_PLACEMENT_3D('',#22212,#15688,#15689);
#14194=AXIS2_PLACEMENT_3D('',#22216,#15692,#15693);
#14195=AXIS2_PLACEMENT_3D('',#22218,#15695,#15696);
#14196=AXIS2_PLACEMENT_3D('',#22219,#15697,#15698);
#14197=AXIS2_PLACEMENT_3D('',#22221,#15700,#15701);
#14198=AXIS2_PLACEMENT_3D('',#22222,#15702,#15703);
#14199=AXIS2_PLACEMENT_3D('',#22224,#15705,#15706);
#14200=AXIS2_PLACEMENT_3D('',#22226,#15708,#15709);
#14201=AXIS2_PLACEMENT_3D('',#22227,#15710,#15711);
#14202=AXIS2_PLACEMENT_3D('',#22229,#15713,#15714);
#14203=AXIS2_PLACEMENT_3D('',#22231,#15716,#15717);
#15455=DIRECTION('axis',(0.,0.,1.));
#15456=DIRECTION('refdir',(1.,0.,0.));
#15457=DIRECTION('center_axis',(0.,0.,1.));
#15458=DIRECTION('ref_axis',(1.,0.,0.));
#15459=DIRECTION('center_axis',(0.,0.,1.));
#15460=DIRECTION('ref_axis',(1.,0.,0.));
#15461=DIRECTION('',(0.707106781186549,8.65956056235495E-17,-0.707106781186546));
#15462=DIRECTION('center_axis',(0.,0.,-1.));
#15463=DIRECTION('ref_axis',(1.,0.,0.));
#15464=DIRECTION('center_axis',(0.,0.,-1.));
#15465=DIRECTION('ref_axis',(1.,0.,0.));
#15466=DIRECTION('',(0.,0.,-1.));
#15467=DIRECTION('center_axis',(0.,0.,1.));
#15468=DIRECTION('ref_axis',(1.,0.,0.));
#15469=DIRECTION('center_axis',(0.,0.,1.));
#15470=DIRECTION('ref_axis',(-1.,0.,0.));
#15471=DIRECTION('',(1.,0.,0.));
#15472=DIRECTION('',(0.,-1.,0.));
#15473=DIRECTION('',(-1.,0.,0.));
#15474=DIRECTION('',(0.,-1.,0.));
#15475=DIRECTION('center_axis',(0.,0.,-1.));
#15476=DIRECTION('ref_axis',(1.,0.,0.));
#15477=DIRECTION('center_axis',(0.,0.,-1.));
#15478=DIRECTION('ref_axis',(1.,0.,0.));
#15479=DIRECTION('',(0.707106781186547,-8.65956056235493E-17,0.707106781186547));
#15480=DIRECTION('center_axis',(0.,0.,-1.));
#15481=DIRECTION('ref_axis',(1.,0.,0.));
#15482=DIRECTION('',(-1.,0.,0.));
#15483=DIRECTION('',(0.,-1.,0.));
#15484=DIRECTION('',(1.,0.,0.));
#15485=DIRECTION('',(0.,-1.,0.));
#15486=DIRECTION('center_axis',(0.,0.707106781186548,0.707106781186547));
#15487=DIRECTION('ref_axis',(1.,0.,0.));
#15488=DIRECTION('',(0.,0.707106781186546,-0.707106781186549));
#15489=DIRECTION('',(-1.,0.,0.));
#15490=DIRECTION('',(1.57009245868377E-15,-0.707106781186547,0.707106781186548));
#15491=DIRECTION('',(1.,0.,0.));
#15492=DIRECTION('center_axis',(0.,1.,0.));
#15493=DIRECTION('ref_axis',(1.,0.,-6.83214169000092E-15));
#15494=DIRECTION('',(0.707106781186546,0.707106781186549,-6.28036983473511E-15));
#15495=DIRECTION('center_axis',(0.,1.,0.));
#15496=DIRECTION('ref_axis',(1.,0.,-6.83214169000092E-15));
#15497=DIRECTION('center_axis',(0.,-1.,0.));
#15498=DIRECTION('ref_axis',(1.,0.,-6.83214169000092E-15));
#15499=DIRECTION('center_axis',(-0.707106781186549,0.707106781186546,0.));
#15500=DIRECTION('ref_axis',(0.,0.,1.));
#15501=DIRECTION('',(0.707106781186546,0.707106781186549,0.));
#15502=DIRECTION('',(0.,0.,-1.));
#15503=DIRECTION('',(0.,0.,1.));
#15504=DIRECTION('center_axis',(0.,1.,0.));
#15505=DIRECTION('ref_axis',(6.83214169000091E-15,0.,1.));
#15506=DIRECTION('',(6.28036983473511E-15,0.707106781186549,0.707106781186546));
#15507=DIRECTION('center_axis',(0.,1.,0.));
#15508=DIRECTION('ref_axis',(6.83214169000091E-15,0.,1.));
#15509=DIRECTION('center_axis',(0.,-1.,0.));
#15510=DIRECTION('ref_axis',(6.83214169000091E-15,0.,1.));
#15511=DIRECTION('center_axis',(0.,0.707106781186548,-0.707106781186547));
#15512=DIRECTION('ref_axis',(-1.,0.,0.));
#15513=DIRECTION('',(0.,0.707106781186547,0.707106781186548));
#15514=DIRECTION('',(1.,0.,0.));
#15515=DIRECTION('center_axis',(0.,1.,0.));
#15516=DIRECTION('ref_axis',(-1.,0.,-1.70803542250024E-15));
#15517=DIRECTION('',(-0.707106781186548,0.707106781186547,0.));
#15518=DIRECTION('center_axis',(0.,1.,0.));
#15519=DIRECTION('ref_axis',(-1.,0.,-1.70803542250024E-15));
#15520=DIRECTION('center_axis',(0.,-1.,0.));
#15521=DIRECTION('ref_axis',(-1.,0.,-1.70803542250024E-15));
#15522=DIRECTION('center_axis',(0.707106781186548,0.707106781186547,0.));
#15523=DIRECTION('ref_axis',(0.,0.,-1.));
#15524=DIRECTION('',(-0.707106781186548,0.707106781186547,0.));
#15525=DIRECTION('',(0.,0.,1.));
#15526=DIRECTION('',(0.,0.,-1.));
#15527=DIRECTION('center_axis',(0.,1.,0.));
#15528=DIRECTION('ref_axis',(0.,0.,-1.));
#15529=DIRECTION('center_axis',(0.,1.,0.));
#15530=DIRECTION('ref_axis',(0.,0.,-1.));
#15531=DIRECTION('center_axis',(0.,-1.,0.));
#15532=DIRECTION('ref_axis',(0.,0.,-1.));
#15533=DIRECTION('center_axis',(0.,-1.,0.));
#15534=DIRECTION('ref_axis',(6.83214169000091E-15,0.,1.));
#15535=DIRECTION('',(0.,-1.,0.));
#15536=DIRECTION('center_axis',(0.,1.,0.));
#15537=DIRECTION('ref_axis',(6.83214169000091E-15,0.,1.));
#15538=DIRECTION('center_axis',(-1.,0.,0.));
#15539=DIRECTION('ref_axis',(0.,0.,-1.));
#15540=DIRECTION('',(0.,-1.,0.));
#15541=DIRECTION('',(0.,0.,-1.));
#15542=DIRECTION('center_axis',(0.,-1.,0.));
#15543=DIRECTION('ref_axis',(1.,0.,-6.83214169000092E-15));
#15544=DIRECTION('',(0.,-1.,0.));
#15545=DIRECTION('center_axis',(0.,1.,0.));
#15546=DIRECTION('ref_axis',(1.,0.,-6.83214169000092E-15));
#15547=DIRECTION('center_axis',(0.,0.,1.));
#15548=DIRECTION('ref_axis',(-1.,0.,0.));
#15549=DIRECTION('',(0.,-1.,0.));
#15550=DIRECTION('',(-1.,0.,0.));
#15551=DIRECTION('center_axis',(0.,1.,0.));
#15552=DIRECTION('ref_axis',(1.,0.,0.));
#15553=DIRECTION('center_axis',(0.,-1.,0.));
#15554=DIRECTION('ref_axis',(1.97372982155583E-15,0.,1.));
#15555=DIRECTION('',(0.,0.,1.));
#15556=DIRECTION('center_axis',(0.,-1.,0.));
#15557=DIRECTION('ref_axis',(1.,0.,-1.97372982155583E-15));
#15558=DIRECTION('',(1.,0.,0.));
#15559=DIRECTION('center_axis',(0.,-1.,0.));
#15560=DIRECTION('ref_axis',(1.2335811384724E-16,0.,-1.));
#15561=DIRECTION('',(0.,0.,-1.));
#15562=DIRECTION('center_axis',(0.,-1.,0.));
#15563=DIRECTION('ref_axis',(-1.,0.,0.));
#15564=DIRECTION('',(-1.,0.,0.));
#15565=DIRECTION('center_axis',(0.,-1.,0.));
#15566=DIRECTION('ref_axis',(1.97372982155583E-15,0.,1.));
#15567=DIRECTION('',(-0.707106781186549,0.707106781186546,-3.14018491736754E-15));
#15568=DIRECTION('',(0.,-0.707106781186549,0.707106781186546));
#15569=DIRECTION('center_axis',(0.,1.,0.));
#15570=DIRECTION('ref_axis',(1.97372982155583E-15,0.,1.));
#15571=DIRECTION('center_axis',(0.707106781186549,0.707106781186546,0.));
#15572=DIRECTION('ref_axis',(0.,0.,-1.));
#15573=DIRECTION('',(0.,0.,-1.));
#15574=DIRECTION('',(-0.707106781186546,0.707106781186549,0.));
#15575=DIRECTION('center_axis',(0.,-1.,0.));
#15576=DIRECTION('ref_axis',(1.,0.,-1.97372982155583E-15));
#15577=DIRECTION('',(0.,0.707106781186549,0.707106781186546));
#15578=DIRECTION('center_axis',(0.,1.,0.));
#15579=DIRECTION('ref_axis',(1.,0.,-1.97372982155583E-15));
#15580=DIRECTION('center_axis',(0.,0.707106781186546,-0.707106781186549));
#15581=DIRECTION('ref_axis',(-1.,0.,0.));
#15582=DIRECTION('',(-1.,0.,0.));
#15583=DIRECTION('',(-7.85046229341889E-16,0.707106781186549,0.707106781186546));
#15584=DIRECTION('center_axis',(0.,-1.,0.));
#15585=DIRECTION('ref_axis',(1.2335811384724E-16,0.,-1.));
#15586=DIRECTION('',(0.707106781186547,0.707106781186548,0.));
#15587=DIRECTION('center_axis',(0.,1.,0.));
#15588=DIRECTION('ref_axis',(1.2335811384724E-16,0.,-1.));
#15589=DIRECTION('center_axis',(-0.707106781186548,0.707106781186547,0.));
#15590=DIRECTION('ref_axis',(0.,0.,1.));
#15591=DIRECTION('',(0.,0.,1.));
#15592=DIRECTION('',(0.707106781186547,0.707106781186548,0.));
#15593=DIRECTION('center_axis',(0.,-1.,0.));
#15594=DIRECTION('ref_axis',(-1.,0.,0.));
#15595=DIRECTION('',(0.,0.707106781186549,-0.707106781186546));
#15596=DIRECTION('center_axis',(0.,1.,0.));
#15597=DIRECTION('ref_axis',(-1.,0.,0.));
#15598=DIRECTION('center_axis',(0.,0.707106781186546,0.707106781186549));
#15599=DIRECTION('ref_axis',(1.,0.,0.));
#15600=DIRECTION('center_axis',(0.,0.,-1.));
#15601=DIRECTION('ref_axis',(1.,0.,0.));
#15602=DIRECTION('',(0.,-1.,0.));
#15603=DIRECTION('',(1.,0.,0.));
#15604=DIRECTION('',(0.,-1.,0.));
#15605=DIRECTION('center_axis',(0.,-1.,0.));
#15606=DIRECTION('ref_axis',(1.,0.,-1.97372982155583E-15));
#15607=DIRECTION('',(0.,-1.,0.));
#15608=DIRECTION('center_axis',(0.,-1.,0.));
#15609=DIRECTION('ref_axis',(1.,0.,-1.97372982155583E-15));
#15610=DIRECTION('center_axis',(1.,0.,0.));
#15611=DIRECTION('ref_axis',(0.,0.,1.));
#15612=DIRECTION('',(0.,-1.,0.));
#15613=DIRECTION('',(0.,0.,1.));
#15614=DIRECTION('center_axis',(0.,-1.,0.));
#15615=DIRECTION('ref_axis',(1.97372982155583E-15,0.,1.));
#15616=DIRECTION('center_axis',(0.,-1.,0.));
#15617=DIRECTION('ref_axis',(1.97372982155583E-15,0.,1.));
#15618=DIRECTION('center_axis',(0.,-0.707106781186548,-0.707106781186548));
#15619=DIRECTION('ref_axis',(-1.,0.,0.));
#15620=DIRECTION('',(0.,-0.707106781186548,0.707106781186548));
#15621=DIRECTION('',(-1.,0.,0.));
#15622=DIRECTION('',(6.54205191118239E-16,0.707106781186548,-0.707106781186548));
#15623=DIRECTION('center_axis',(0.,1.,0.));
#15624=DIRECTION('ref_axis',(1.,0.,-1.97372982155583E-15));
#15625=DIRECTION('',(-0.70710678118655,-0.707106781186545,2.61682076447295E-15));
#15626=DIRECTION('center_axis',(0.,1.,0.));
#15627=DIRECTION('ref_axis',(1.,0.,-1.97372982155583E-15));
#15628=DIRECTION('center_axis',(0.707106781186548,-0.707106781186548,0.));
#15629=DIRECTION('ref_axis',(0.,0.,-1.));
#15630=DIRECTION('',(-0.707106781186548,-0.707106781186548,2.61682076447296E-15));
#15631=DIRECTION('',(0.,0.,-1.));
#15632=DIRECTION('center_axis',(0.,1.,0.));
#15633=DIRECTION('ref_axis',(1.97372982155583E-15,0.,1.));
#15634=DIRECTION('',(0.,-0.707106781186545,-0.70710678118655));
#15635=DIRECTION('center_axis',(0.,1.,0.));
#15636=DIRECTION('ref_axis',(1.97372982155583E-15,0.,1.));
#15637=DIRECTION('center_axis',(0.,-0.707106781186548,0.707106781186548));
#15638=DIRECTION('ref_axis',(1.,0.,0.));
#15639=DIRECTION('',(-1.96261557335472E-15,-0.707106781186548,-0.707106781186548));
#15640=DIRECTION('',(1.,0.,0.));
#15641=DIRECTION('center_axis',(0.,1.,0.));
#15642=DIRECTION('ref_axis',(-1.,0.,0.));
#15643=DIRECTION('',(0.707106781186548,-0.707106781186547,0.));
#15644=DIRECTION('center_axis',(0.,1.,0.));
#15645=DIRECTION('ref_axis',(-1.,0.,0.));
#15646=DIRECTION('center_axis',(0.,-1.,0.));
#15647=DIRECTION('ref_axis',(-1.,0.,0.));
#15648=DIRECTION('center_axis',(-0.707106781186549,-0.707106781186546,0.));
#15649=DIRECTION('ref_axis',(0.,0.,1.));
#15650=DIRECTION('',(0.707106781186546,-0.707106781186549,-2.61682076447296E-15));
#15651=DIRECTION('',(0.,0.,1.));
#15652=DIRECTION('',(0.,0.,-1.));
#15653=DIRECTION('center_axis',(0.,1.,0.));
#15654=DIRECTION('ref_axis',(1.2335811384724E-16,0.,-1.));
#15655=DIRECTION('center_axis',(0.,1.,0.));
#15656=DIRECTION('ref_axis',(1.2335811384724E-16,0.,-1.));
#15657=DIRECTION('center_axis',(0.,-1.,0.));
#15658=DIRECTION('ref_axis',(1.2335811384724E-16,0.,-1.));
#15659=DIRECTION('center_axis',(0.,1.,0.));
#15660=DIRECTION('ref_axis',(1.,0.,0.));
#15661=DIRECTION('',(0.,0.,1.));
#15662=DIRECTION('center_axis',(0.,-1.,0.));
#15663=DIRECTION('ref_axis',(1.,0.,-6.83214169000092E-15));
#15664=DIRECTION('',(1.,0.,0.));
#15665=DIRECTION('center_axis',(0.,-1.,0.));
#15666=DIRECTION('ref_axis',(0.,0.,-1.));
#15667=DIRECTION('',(0.,0.,-1.));
#15668=DIRECTION('center_axis',(0.,-1.,0.));
#15669=DIRECTION('ref_axis',(-1.,0.,-1.70803542250024E-15));
#15670=DIRECTION('',(-1.,0.,0.));
#15671=DIRECTION('center_axis',(0.,-1.,0.));
#15672=DIRECTION('ref_axis',(6.83214169000091E-15,0.,1.));
#15673=DIRECTION('center_axis',(-0.707106781186548,-0.707106781186548,0.));
#15674=DIRECTION('ref_axis',(0.,0.,1.));
#15675=DIRECTION('',(0.707106781186548,-0.707106781186548,-2.61682076447296E-15));
#15676=DIRECTION('',(-0.707106781186548,0.707106781186548,0.));
#15677=DIRECTION('center_axis',(0.,-1.,0.));
#15678=DIRECTION('ref_axis',(1.,0.,-6.83214169000092E-15));
#15679=DIRECTION('',(5.23364152894591E-15,-0.707106781186548,-0.707106781186548));
#15680=DIRECTION('center_axis',(0.,-0.707106781186548,0.707106781186548));
#15681=DIRECTION('ref_axis',(1.,0.,0.));
#15682=DIRECTION('',(-1.30841038223648E-15,-0.707106781186548,-0.707106781186548));
#15683=DIRECTION('center_axis',(0.,-1.,0.));
#15684=DIRECTION('ref_axis',(0.,0.,-1.));
#15685=DIRECTION('',(-0.707106781186547,-0.707106781186548,0.));
#15686=DIRECTION('center_axis',(0.,1.,0.));
#15687=DIRECTION('ref_axis',(0.,0.,-1.));
#15688=DIRECTION('center_axis',(0.707106781186548,-0.707106781186548,0.));
#15689=DIRECTION('ref_axis',(0.,0.,-1.));
#15690=DIRECTION('',(-0.707106781186548,-0.707106781186548,2.61682076447296E-15));
#15691=DIRECTION('',(0.,0.,1.));
#15692=DIRECTION('center_axis',(0.,-1.,0.));
#15693=DIRECTION('ref_axis',(-1.,0.,-1.70803542250024E-15));
#15694=DIRECTION('',(0.,-0.707106781186548,0.707106781186548));
#15695=DIRECTION('center_axis',(0.,1.,0.));
#15696=DIRECTION('ref_axis',(-1.,0.,-1.70803542250024E-15));
#15697=DIRECTION('center_axis',(0.,-0.707106781186548,-0.707106781186548));
#15698=DIRECTION('ref_axis',(-1.,0.,0.));
#15699=DIRECTION('',(0.,-0.707106781186548,0.707106781186548));
#15700=DIRECTION('center_axis',(0.,-1.,0.));
#15701=DIRECTION('ref_axis',(6.83214169000091E-15,0.,1.));
#15702=DIRECTION('center_axis',(0.,-1.,0.));
#15703=DIRECTION('ref_axis',(0.,0.,-1.));
#15704=DIRECTION('',(0.,-1.,0.));
#15705=DIRECTION('center_axis',(0.,-1.,0.));
#15706=DIRECTION('ref_axis',(-1.,0.,-1.70803542250024E-15));
#15707=DIRECTION('',(0.,-1.,0.));
#15708=DIRECTION('center_axis',(1.,0.,0.));
#15709=DIRECTION('ref_axis',(0.,0.,1.));
#15710=DIRECTION('center_axis',(0.,-1.,0.));
#15711=DIRECTION('ref_axis',(1.2335811384724E-16,0.,-1.));
#15712=DIRECTION('',(0.,-1.,0.));
#15713=DIRECTION('center_axis',(-1.,0.,0.));
#15714=DIRECTION('ref_axis',(0.,0.,-1.));
#15715=DIRECTION('',(0.,-1.,0.));
#15716=DIRECTION('center_axis',(0.,-1.,0.));
#15717=DIRECTION('ref_axis',(-1.,0.,0.));
#21991=CARTESIAN_POINT('',(0.,0.,0.));
#21992=CARTESIAN_POINT('Origin',(15.2,-16.,21.975));
#21993=CARTESIAN_POINT('',(12.25,-16.,22.225));
#21994=CARTESIAN_POINT('Origin',(15.2,-16.,22.225));
#21995=CARTESIAN_POINT('',(12.75,-16.,21.725));
#21996=CARTESIAN_POINT('',(12.5,-16.,21.975));
#21997=CARTESIAN_POINT('Origin',(15.2,-16.,21.725));
#21998=CARTESIAN_POINT('Origin',(15.2,-16.,22.225));
#21999=CARTESIAN_POINT('',(12.75,-16.,19.525));
#22000=CARTESIAN_POINT('',(12.75,-16.,22.225));
#22001=CARTESIAN_POINT('Origin',(15.2,-16.,19.525));
#22002=CARTESIAN_POINT('Origin',(32.925,0.,22.225));
#22003=CARTESIAN_POINT('',(-2.525,-0.5,22.225));
#22004=CARTESIAN_POINT('',(32.925,-0.5,22.225));
#22005=CARTESIAN_POINT('',(24.0625,-0.5,22.225));
#22006=CARTESIAN_POINT('',(-2.525,-31.15,22.225));
#22007=CARTESIAN_POINT('',(-2.525,0.,22.225));
#22008=CARTESIAN_POINT('',(32.925,-31.15,22.225));
#22009=CARTESIAN_POINT('',(24.0625,-31.15,22.225));
#22010=CARTESIAN_POINT('',(32.925,0.,22.225));
#22011=CARTESIAN_POINT('Origin',(15.2,-16.,19.275));
#22012=CARTESIAN_POINT('',(12.25,-16.,19.025));
#22013=CARTESIAN_POINT('Origin',(15.2,-16.,19.025));
#22014=CARTESIAN_POINT('',(12.5,-16.,19.275));
#22015=CARTESIAN_POINT('Origin',(-2.525,0.,19.025));
#22016=CARTESIAN_POINT('',(32.925,-0.5,19.025));
#22017=CARTESIAN_POINT('',(-2.525,-0.5,19.025));
#22018=CARTESIAN_POINT('',(6.3375,-0.5,19.025));
#22019=CARTESIAN_POINT('',(32.925,-31.15,19.025));
#22020=CARTESIAN_POINT('',(32.925,0.,19.025));
#22021=CARTESIAN_POINT('',(-2.525,-31.15,19.025));
#22022=CARTESIAN_POINT('',(6.3375,-31.15,19.025));
#22023=CARTESIAN_POINT('',(-2.525,0.,19.025));
#22024=CARTESIAN_POINT('Origin',(24.0625,-0.25,-19.275));
#22025=CARTESIAN_POINT('',(32.925,-0.5,-19.025));
#22026=CARTESIAN_POINT('',(32.925,0.,-19.525));
#22027=CARTESIAN_POINT('',(32.925,-0.5,-19.025));
#22028=CARTESIAN_POINT('',(-2.525,0.,-19.525));
#22029=CARTESIAN_POINT('',(24.0625,0.,-19.525));
#22030=CARTESIAN_POINT('',(-2.525,-0.5,-19.025));
#22031=CARTESIAN_POINT('',(-2.525,0.,-19.525));
#22032=CARTESIAN_POINT('',(24.0625,-0.5,-19.025));
#22033=CARTESIAN_POINT('Origin',(32.925,-0.25,-17.725));
#22034=CARTESIAN_POINT('',(34.225,-0.5,-17.725));
#22035=CARTESIAN_POINT('',(34.725,0.,-17.725));
#22036=CARTESIAN_POINT('',(34.225,-0.5,-17.725));
#22037=CARTESIAN_POINT('Origin',(32.925,0.,-17.725));
#22038=CARTESIAN_POINT('Origin',(32.925,-0.5,-17.725));
#22039=CARTESIAN_POINT('Origin',(34.475,-0.25,8.8625));
#22040=CARTESIAN_POINT('',(34.225,-0.5,17.725));
#22041=CARTESIAN_POINT('',(34.725,0.,17.725));
#22042=CARTESIAN_POINT('',(34.225,-0.5,17.725));
#22043=CARTESIAN_POINT('',(34.725,0.,8.8625));
#22044=CARTESIAN_POINT('',(34.225,-0.5,8.8625));
#22045=CARTESIAN_POINT('Origin',(32.925,-0.25,17.725));
#22046=CARTESIAN_POINT('',(32.925,0.,19.525));
#22047=CARTESIAN_POINT('',(32.925,-0.5,19.025));
#22048=CARTESIAN_POINT('Origin',(32.925,0.,17.725));
#22049=CARTESIAN_POINT('Origin',(32.925,-0.5,17.725));
#22050=CARTESIAN_POINT('Origin',(6.3375,-0.25,19.275));
#22051=CARTESIAN_POINT('',(-2.525,0.,19.525));
#22052=CARTESIAN_POINT('',(-2.525,-0.5,19.025));
#22053=CARTESIAN_POINT('',(6.3375,0.,19.525));
#22054=CARTESIAN_POINT('Origin',(-2.525,-0.25,17.725));
#22055=CARTESIAN_POINT('',(-3.825,-0.5,17.725));
#22056=CARTESIAN_POINT('',(-4.325,0.,17.725));
#22057=CARTESIAN_POINT('',(-3.825,-0.5,17.725));
#22058=CARTESIAN_POINT('Origin',(-2.525,0.,17.725));
#22059=CARTESIAN_POINT('Origin',(-2.525,-0.5,17.725));
#22060=CARTESIAN_POINT('Origin',(-4.075,-0.25,-8.8625));
#22061=CARTESIAN_POINT('',(-3.825,-0.5,-17.725));
#22062=CARTESIAN_POINT('',(-4.325,0.,-17.725));
#22063=CARTESIAN_POINT('',(-3.825,-0.5,-17.725));
#22064=CARTESIAN_POINT('',(-4.325,0.,-8.8625));
#22065=CARTESIAN_POINT('',(-3.825,-0.5,-8.8625));
#22066=CARTESIAN_POINT('Origin',(-2.525,-0.25,-17.725));
#22067=CARTESIAN_POINT('Origin',(-2.525,0.,-17.725));
#22068=CARTESIAN_POINT('Origin',(-2.525,-0.5,-17.725));
#22069=CARTESIAN_POINT('Origin',(32.925,0.,17.725));
#22070=CARTESIAN_POINT('',(34.225,-31.15,17.725));
#22071=CARTESIAN_POINT('',(34.225,0.,17.725));
#22072=CARTESIAN_POINT('Origin',(32.925,-31.15,17.725));
#22073=CARTESIAN_POINT('Origin',(34.225,0.,17.725));
#22074=CARTESIAN_POINT('',(34.225,-31.15,-17.725));
#22075=CARTESIAN_POINT('',(34.225,0.,-17.725));
#22076=CARTESIAN_POINT('',(34.225,-31.15,8.8625));
#22077=CARTESIAN_POINT('Origin',(32.925,0.,-17.725));
#22078=CARTESIAN_POINT('',(32.925,-31.15,-19.025));
#22079=CARTESIAN_POINT('',(32.925,0.,-19.025));
#22080=CARTESIAN_POINT('Origin',(32.925,-31.15,-17.725));
#22081=CARTESIAN_POINT('Origin',(32.925,0.,-19.025));
#22082=CARTESIAN_POINT('',(-2.525,-31.15,-19.025));
#22083=CARTESIAN_POINT('',(-2.525,0.,-19.025));
#22084=CARTESIAN_POINT('',(24.0625,-31.15,-19.025));
#22085=CARTESIAN_POINT('Origin',(15.2,0.,0.));
#22086=CARTESIAN_POINT('',(36.925,0.,17.725));
#22087=CARTESIAN_POINT('',(32.925,0.,21.725));
#22088=CARTESIAN_POINT('Origin',(32.925,0.,17.725));
#22089=CARTESIAN_POINT('',(36.925,0.,-17.725));
#22090=CARTESIAN_POINT('',(36.925,0.,-8.8625));
#22091=CARTESIAN_POINT('',(32.925,0.,-21.725));
#22092=CARTESIAN_POINT('Origin',(32.925,0.,-17.725));
#22093=CARTESIAN_POINT('',(-2.525,0.,-21.725));
#22094=CARTESIAN_POINT('',(6.3375,0.,-21.725));
#22095=CARTESIAN_POINT('',(-6.525,0.,-17.725));
#22096=CARTESIAN_POINT('Origin',(-2.525,0.,-17.725));
#22097=CARTESIAN_POINT('',(-6.525,0.,17.725));
#22098=CARTESIAN_POINT('',(-6.525,0.,8.8625));
#22099=CARTESIAN_POINT('',(-2.525,0.,21.725));
#22100=CARTESIAN_POINT('Origin',(-2.525,0.,17.725));
#22101=CARTESIAN_POINT('',(24.0625,0.,21.725));
#22102=CARTESIAN_POINT('Origin',(32.925,-0.25,17.725));
#22103=CARTESIAN_POINT('',(37.425,-0.5,17.725));
#22104=CARTESIAN_POINT('',(37.425,-0.5,17.725));
#22105=CARTESIAN_POINT('',(32.925,0.,21.725));
#22106=CARTESIAN_POINT('Origin',(32.925,-0.5,17.725));
#22107=CARTESIAN_POINT('Origin',(37.175,-0.25,-8.8625));
#22108=CARTESIAN_POINT('',(37.425,-0.5,-17.725));
#22109=CARTESIAN_POINT('',(37.425,-0.5,-8.8625));
#22110=CARTESIAN_POINT('',(37.425,-0.5,-17.725));
#22111=CARTESIAN_POINT('Origin',(32.925,-0.25,-17.725));
#22112=CARTESIAN_POINT('',(32.925,-0.5,-22.225));
#22113=CARTESIAN_POINT('',(32.925,-0.5,-22.225));
#22114=CARTESIAN_POINT('Origin',(32.925,-0.5,-17.725));
#22115=CARTESIAN_POINT('Origin',(6.3375,-0.25,-21.975));
#22116=CARTESIAN_POINT('',(-2.525,-0.5,-22.225));
#22117=CARTESIAN_POINT('',(6.3375,-0.5,-22.225));
#22118=CARTESIAN_POINT('',(-2.525,-0.5,-22.225));
#22119=CARTESIAN_POINT('Origin',(-2.525,-0.25,-17.725));
#22120=CARTESIAN_POINT('',(-7.025,-0.5,-17.725));
#22121=CARTESIAN_POINT('',(-7.025,-0.5,-17.725));
#22122=CARTESIAN_POINT('Origin',(-2.525,-0.5,-17.725));
#22123=CARTESIAN_POINT('Origin',(-6.775,-0.25,8.8625));
#22124=CARTESIAN_POINT('',(-7.025,-0.5,17.725));
#22125=CARTESIAN_POINT('',(-7.025,-0.5,8.8625));
#22126=CARTESIAN_POINT('',(-7.025,-0.5,17.725));
#22127=CARTESIAN_POINT('Origin',(-2.525,-0.25,17.725));
#22128=CARTESIAN_POINT('',(-2.525,-0.5,22.225));
#22129=CARTESIAN_POINT('Origin',(-2.525,-0.5,17.725));
#22130=CARTESIAN_POINT('Origin',(24.0625,-0.25,21.975));
#22131=CARTESIAN_POINT('Origin',(-2.525,0.,-22.225));
#22132=CARTESIAN_POINT('',(32.925,-31.15,-22.225));
#22133=CARTESIAN_POINT('',(32.925,0.,-22.225));
#22134=CARTESIAN_POINT('',(-2.525,-31.15,-22.225));
#22135=CARTESIAN_POINT('',(6.3375,-31.15,-22.225));
#22136=CARTESIAN_POINT('',(-2.525,0.,-22.225));
#22137=CARTESIAN_POINT('Origin',(32.925,0.,-17.725));
#22138=CARTESIAN_POINT('',(37.425,-31.15,-17.725));
#22139=CARTESIAN_POINT('',(37.425,0.,-17.725));
#22140=CARTESIAN_POINT('Origin',(32.925,-31.15,-17.725));
#22141=CARTESIAN_POINT('Origin',(37.425,0.,-17.725));
#22142=CARTESIAN_POINT('',(37.425,-31.15,17.725));
#22143=CARTESIAN_POINT('',(37.425,0.,17.725));
#22144=CARTESIAN_POINT('',(37.425,-31.15,-8.8625));
#22145=CARTESIAN_POINT('Origin',(32.925,0.,17.725));
#22146=CARTESIAN_POINT('Origin',(32.925,-31.15,17.725));
#22147=CARTESIAN_POINT('Origin',(6.3375,-31.45,-21.925));
#22148=CARTESIAN_POINT('',(32.925,-31.75,-21.625));
#22149=CARTESIAN_POINT('',(32.925,-31.15,-22.225));
#22150=CARTESIAN_POINT('',(-2.525,-31.75,-21.625));
#22151=CARTESIAN_POINT('',(6.3375,-31.75,-21.625));
#22152=CARTESIAN_POINT('',(-2.525,-31.75,-21.625));
#22153=CARTESIAN_POINT('Origin',(32.925,-31.45,-17.725));
#22154=CARTESIAN_POINT('',(36.825,-31.75,-17.725));
#22155=CARTESIAN_POINT('',(37.425,-31.15,-17.725));
#22156=CARTESIAN_POINT('Origin',(32.925,-31.75,-17.725));
#22157=CARTESIAN_POINT('Origin',(37.125,-31.45,-8.8625));
#22158=CARTESIAN_POINT('',(36.825,-31.75,17.725));
#22159=CARTESIAN_POINT('',(37.425,-31.15,17.725));
#22160=CARTESIAN_POINT('',(36.825,-31.75,-8.8625));
#22161=CARTESIAN_POINT('Origin',(32.925,-31.45,17.725));
#22162=CARTESIAN_POINT('',(32.925,-31.75,21.625));
#22163=CARTESIAN_POINT('',(32.925,-31.15,22.225));
#22164=CARTESIAN_POINT('Origin',(32.925,-31.75,17.725));
#22165=CARTESIAN_POINT('Origin',(24.0625,-31.45,21.925));
#22166=CARTESIAN_POINT('',(-2.525,-31.75,21.625));
#22167=CARTESIAN_POINT('',(-2.525,-31.15,22.225));
#22168=CARTESIAN_POINT('',(24.0625,-31.75,21.625));
#22169=CARTESIAN_POINT('Origin',(-2.525,-31.45,17.725));
#22170=CARTESIAN_POINT('',(-7.025,-31.15,17.725));
#22171=CARTESIAN_POINT('',(-6.425,-31.75,17.725));
#22172=CARTESIAN_POINT('',(-7.025,-31.15,17.725));
#22173=CARTESIAN_POINT('Origin',(-2.525,-31.75,17.725));
#22174=CARTESIAN_POINT('Origin',(-2.525,-31.15,17.725));
#22175=CARTESIAN_POINT('Origin',(-6.725,-31.45,8.8625));
#22176=CARTESIAN_POINT('',(-7.025,-31.15,-17.725));
#22177=CARTESIAN_POINT('',(-6.425,-31.75,-17.725));
#22178=CARTESIAN_POINT('',(-7.025,-31.15,-17.725));
#22179=CARTESIAN_POINT('',(-6.425,-31.75,8.8625));
#22180=CARTESIAN_POINT('',(-7.025,-31.15,8.8625));
#22181=CARTESIAN_POINT('Origin',(-2.525,-31.45,-17.725));
#22182=CARTESIAN_POINT('Origin',(-2.525,-31.75,-17.725));
#22183=CARTESIAN_POINT('Origin',(-2.525,-31.15,-17.725));
#22184=CARTESIAN_POINT('Origin',(15.2,-31.75,0.));
#22185=CARTESIAN_POINT('',(34.825,-31.75,-17.725));
#22186=CARTESIAN_POINT('',(34.825,-31.75,17.725));
#22187=CARTESIAN_POINT('',(34.825,-31.75,8.8625));
#22188=CARTESIAN_POINT('',(32.925,-31.75,-19.625));
#22189=CARTESIAN_POINT('Origin',(32.925,-31.75,-17.725));
#22190=CARTESIAN_POINT('',(-2.525,-31.75,-19.625));
#22191=CARTESIAN_POINT('',(24.0625,-31.75,-19.625));
#22192=CARTESIAN_POINT('',(-4.425,-31.75,-17.725));
#22193=CARTESIAN_POINT('Origin',(-2.525,-31.75,-17.725));
#22194=CARTESIAN_POINT('',(-4.425,-31.75,17.725));
#22195=CARTESIAN_POINT('',(-4.425,-31.75,-8.8625));
#22196=CARTESIAN_POINT('',(-2.525,-31.75,19.625));
#22197=CARTESIAN_POINT('Origin',(-2.525,-31.75,17.725));
#22198=CARTESIAN_POINT('',(32.925,-31.75,19.625));
#22199=CARTESIAN_POINT('',(6.3375,-31.75,19.625));
#22200=CARTESIAN_POINT('Origin',(32.925,-31.75,17.725));
#22201=CARTESIAN_POINT('Origin',(34.525,-31.45,8.8625));
#22202=CARTESIAN_POINT('',(34.225,-31.15,-17.725));
#22203=CARTESIAN_POINT('',(34.825,-31.75,17.725));
#22204=CARTESIAN_POINT('Origin',(32.925,-31.45,-17.725));
#22205=CARTESIAN_POINT('',(32.925,-31.15,-19.025));
#22206=CARTESIAN_POINT('Origin',(24.0625,-31.45,-19.325));
#22207=CARTESIAN_POINT('',(-2.525,-31.15,-19.025));
#22208=CARTESIAN_POINT('Origin',(-2.525,-31.45,-17.725));
#22209=CARTESIAN_POINT('',(-3.825,-31.15,-17.725));
#22210=CARTESIAN_POINT('',(-3.825,-31.15,-17.725));
#22211=CARTESIAN_POINT('Origin',(-2.525,-31.15,-17.725));
#22212=CARTESIAN_POINT('Origin',(-4.125,-31.45,-8.8625));
#22213=CARTESIAN_POINT('',(-3.825,-31.15,17.725));
#22214=CARTESIAN_POINT('',(-3.825,-31.15,17.725));
#22215=CARTESIAN_POINT('',(-3.825,-31.15,-8.8625));
#22216=CARTESIAN_POINT('Origin',(-2.525,-31.45,17.725));
#22217=CARTESIAN_POINT('',(-2.525,-31.15,19.025));
#22218=CARTESIAN_POINT('Origin',(-2.525,-31.15,17.725));
#22219=CARTESIAN_POINT('Origin',(6.3375,-31.45,19.325));
#22220=CARTESIAN_POINT('',(32.925,-31.15,19.025));
#22221=CARTESIAN_POINT('Origin',(32.925,-31.45,17.725));
#22222=CARTESIAN_POINT('Origin',(-2.525,0.,-17.725));
#22223=CARTESIAN_POINT('',(-3.825,0.,-17.725));
#22224=CARTESIAN_POINT('Origin',(-2.525,0.,17.725));
#22225=CARTESIAN_POINT('',(-3.825,0.,17.725));
#22226=CARTESIAN_POINT('Origin',(-3.825,0.,-17.725));
#22227=CARTESIAN_POINT('Origin',(-2.525,0.,-17.725));
#22228=CARTESIAN_POINT('',(-7.025,0.,-17.725));
#22229=CARTESIAN_POINT('Origin',(-7.025,0.,17.725));
#22230=CARTESIAN_POINT('',(-7.025,0.,17.725));
#22231=CARTESIAN_POINT('Origin',(-2.525,0.,17.725));
#32282=UNCERTAINTY_MEASURE_WITH_UNIT(LENGTH_MEASURE(0.01),#32310,
'DISTANCE_ACCURACY_VALUE',
'Maximum model space distance between geometric entities at asserted c
onnectivities');
#32293=UNCERTAINTY_MEASURE_WITH_UNIT(LENGTH_MEASURE(0.01),#32310,
'DISTANCE_ACCURACY_VALUE',
'Maximum model space distance between geometric entities at asserted c
onnectivities');
#32298=(
GEOMETRIC_REPRESENTATION_CONTEXT(3)
GLOBAL_UNCERTAINTY_ASSIGNED_CONTEXT((#32282))
GLOBAL_UNIT_ASSIGNED_CONTEXT((#32310,#32312,#32313))
REPRESENTATION_CONTEXT('','3D')
);
#32309=(
GEOMETRIC_REPRESENTATION_CONTEXT(3)
GLOBAL_UNCERTAINTY_ASSIGNED_CONTEXT((#32293))
GLOBAL_UNIT_ASSIGNED_CONTEXT((#32310,#32312,#32313))
REPRESENTATION_CONTEXT('','3D')
);
#32310=(
LENGTH_UNIT()
NAMED_UNIT(*)
SI_UNIT(.MILLI.,.METRE.)
);
#32312=(
NAMED_UNIT(*)
PLANE_ANGLE_UNIT()
SI_UNIT($,.RADIAN.)
);
#32313=(
NAMED_UNIT(*)
SI_UNIT($,.STERADIAN.)
SOLID_ANGLE_UNIT()
);
#32318=SHAPE_DEFINITION_REPRESENTATION(#32333,#32365);
#32333=PRODUCT_DEFINITION_SHAPE('',$,#32381);
#32365=SHAPE_REPRESENTATION('',(#14114),#32298);
#32376=PRODUCT_DEFINITION_CONTEXT('part definition',#32423,'design');
#32381=PRODUCT_DEFINITION('2026-10-25-00-35-16-238',
'04_Lock_Receiver_1.75sq',#32396,#32376);
#32396=PRODUCT_DEFINITION_FORMATION('',$,#32429);
#32423=APPLICATION_CONTEXT(
'Core Data for Automotive Mechanical Design Process');
#32424=PRODUCT_CONTEXT('part definition',#32423,'mechanical');
#32429=PRODUCT('2026-10-25-00-35-16-238','04_Lock_Receiver_1.75sq',$,(#32424));
#32510=COLOUR_RGB('Off White',0.89,0.88,0.83);
#32511=FILL_AREA_STYLE_COLOUR('',#32510);
#32512=FILL_AREA_STYLE('',(#32511));
#32513=SURFACE_STYLE_FILL_AREA(#32512);
#32514=SURFACE_SIDE_STYLE('',(#32513));
#32515=SURFACE_STYLE_USAGE(.BOTH.,#32514);
#32516=PRESENTATION_STYLE_ASSIGNMENT((#32515));
ENDSEC;
END-ISO-10303-21;
